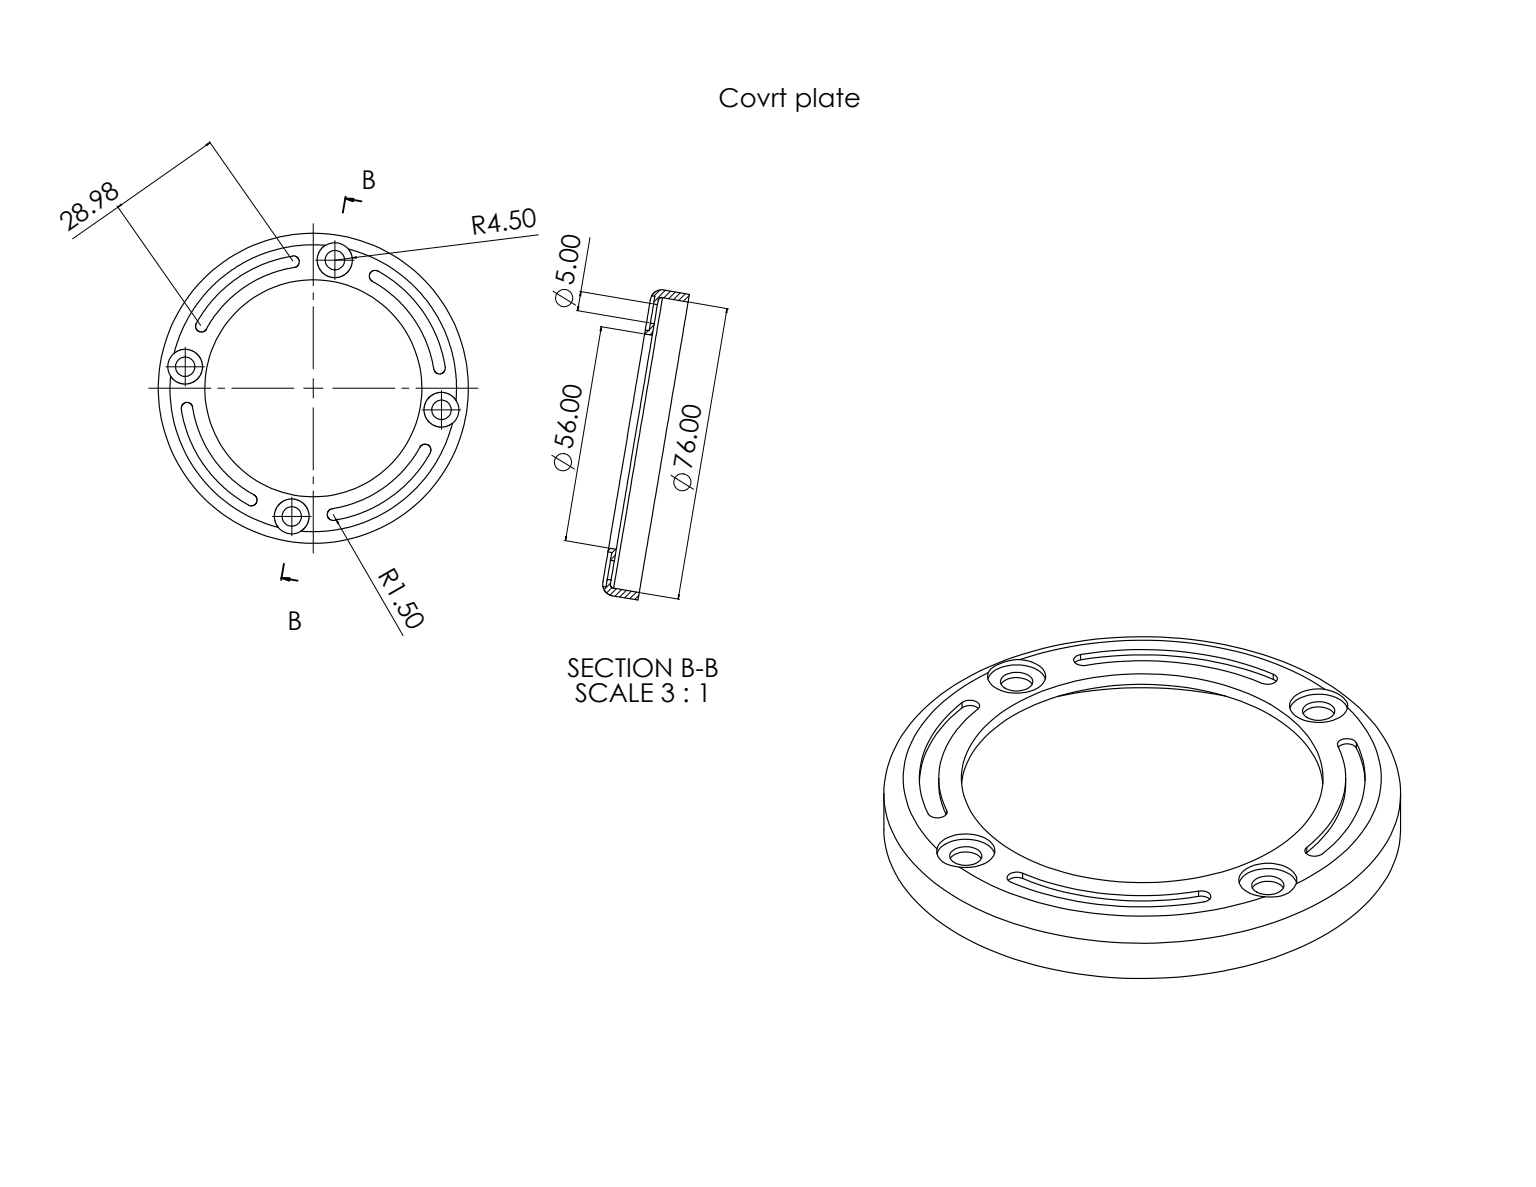
ISO-10303-21;
HEADER;
FILE_DESCRIPTION (('STEP AP214'),
    '1' );
FILE_NAME ('Covrt plate.step',
    '2026-10-19T14:05:14',
    ( '' ),
    ( '' ),
    'SwSTEP 2.0',
    'SolidWorks 2025',
    '' );
FILE_SCHEMA (( 'AUTOMOTIVE_DESIGN' ));
ENDSEC;

DATA;
#7=DIRECTION ( 'NONE',  ( 0.000000000000000000, 0.000000000000000000, 1.000000000000000000 ) ) ;
#9=ORIENTED_EDGE ( 'NONE', *, *, #8476, .T. ) ;
#15=ORIENTED_EDGE ( 'NONE', *, *, #6125, .T. ) ;
#19=DIRECTION ( 'NONE',  ( 0.000000000000000000, 0.000000000000000000, 1.000000000000000000 ) ) ;
#32=ORIENTED_EDGE ( 'NONE', *, *, #3378, .T. ) ;
#35=EDGE_CURVE ( 'NONE', #8414, #7328, #2773, .T. ) ;
#36=ORIENTED_EDGE ( 'NONE', *, *, #1808, .T. ) ;
#37=CARTESIAN_POINT ( 'NONE',  ( -7.819489076939736272, 61.89591950820473443, 36.97167050927867393 ) ) ;
#41=EDGE_CURVE ( 'NONE', #3849, #2645, #7411, .T. ) ;
#45=ORIENTED_EDGE ( 'NONE', *, *, #2688, .T. ) ;
#51=EDGE_CURVE ( 'NONE', #326, #7682, #6952, .T. ) ;
#56=CIRCLE ( 'NONE', #3832, 38.00000000000000711 ) ;
#57=EDGE_LOOP ( 'NONE', ( #2932, #7865, #7571, #5966, #8095 ) ) ;
#58=DIRECTION ( 'NONE',  ( 0.000000000000000000, 1.000000000000000000, 0.000000000000000000 ) ) ;
#64=VERTEX_POINT ( 'NONE', #213 ) ;
#66=LINE ( 'NONE', #799, #8451 ) ;
#76=AXIS2_PLACEMENT_3D ( 'NONE', #8734, #591, #7241 ) ;
#80=ORIENTED_EDGE ( 'NONE', *, *, #3650, .T. ) ;
#85=AXIS2_PLACEMENT_3D ( 'NONE', #944, #4059, #1772 ) ;
#88=ORIENTED_EDGE ( 'NONE', *, *, #8502, .F. ) ;
#89=CARTESIAN_POINT ( 'NONE',  ( 5.562309845534588959, 60.99999999999999289, -30.56426808735054479 ) ) ;
#98=CARTESIAN_POINT ( 'NONE',  ( -34.07933880998930221, 60.99999999999999289, 5.371095444502539173 ) ) ;
#116=DIRECTION ( 'NONE',  ( -0.000000000000000000, -1.000000000000000000, -0.000000000000000000 ) ) ;
#124=DIRECTION ( 'NONE',  ( 0.000000000000000000, 0.000000000000000000, 1.000000000000000000 ) ) ;
#126=CARTESIAN_POINT ( 'NONE',  ( -28.87459861216645862, 60.99999999999999289, -14.47678174684361352 ) ) ;
#129=LINE ( 'NONE', #4464, #7033 ) ;
#133=CARTESIAN_POINT ( 'NONE',  ( -5.562309845534701758, 60.99999999999999289, 33.06426808735052703 ) ) ;
#144=FACE_OUTER_BOUND ( 'NONE', #5084, .T. ) ;
#153=ORIENTED_EDGE ( 'NONE', *, *, #7147, .T. ) ;
#155=CARTESIAN_POINT ( 'NONE',  ( 37.34143203299149860, 61.94837758590841759, 4.137096292553819055 ) ) ;
#162=DIRECTION ( 'NONE',  ( 0.000000000000000000, 0.000000000000000000, 1.000000000000000000 ) ) ;
#168=FACE_OUTER_BOUND ( 'NONE', #440, .T. ) ;
#172=CIRCLE ( 'NONE', #6452, 38.00000000000000711 ) ;
#175=FACE_OUTER_BOUND ( 'NONE', #2105, .T. ) ;
#184=CARTESIAN_POINT ( 'NONE',  ( 31.11591804390324612, 60.99999999999999289, -4.904043666719942074 ) ) ;
#189=ORIENTED_EDGE ( 'NONE', *, *, #8556, .F. ) ;
#198=CIRCLE ( 'NONE', #6955, 4.500000000000005329 ) ;
#200=DIRECTION ( 'NONE',  ( 0.000000000000000000, 0.000000000000000000, 1.000000000000000000 ) ) ;
#203=DIRECTION ( 'NONE',  ( 0.000000000000000000, 0.000000000000000000, 1.000000000000000000 ) ) ;
#211=AXIS2_PLACEMENT_3D ( 'NONE', #6008, #116, #5285 ) ;
#213=CARTESIAN_POINT ( 'NONE',  ( 4.653657836759942730E-15, 52.29648987751954792, 38.00000000000000711 ) ) ;
#216=CARTESIAN_POINT ( 'NONE',  ( 3.429011037612588487E-15, 0.000000000000000000, 27.99999999999999289 ) ) ;
#222=CIRCLE ( 'NONE', #6654, 1.500000000000000888 ) ;
#224=EDGE_CURVE ( 'NONE', #6202, #6468, #9617, .T. ) ;
#225=CIRCLE ( 'NONE', #5729, 4.500000000000005329 ) ;
#239=DIRECTION ( 'NONE',  ( 0.000000000000000000, 1.000000000000000000, 0.000000000000000000 ) ) ;
#241=CARTESIAN_POINT ( 'NONE',  ( 0.000000000000000000, 60.99999999999999289, 0.000000000000000000 ) ) ;
#242=DIRECTION ( 'NONE',  ( 0.000000000000000000, 0.000000000000000000, -1.000000000000000000 ) ) ;
#245=AXIS2_PLACEMENT_3D ( 'NONE', #2886, #4538, #6229 ) ;
#246=CYLINDRICAL_SURFACE ( 'NONE', #7429, 1.500000000000001332 ) ;
#249=EDGE_CURVE ( 'NONE', #5097, #3498, #5520, .T. ) ;
#251=DIRECTION ( 'NONE',  ( 0.000000000000000000, 1.000000000000000000, 0.000000000000000000 ) ) ;
#256=ORIENTED_EDGE ( 'NONE', *, *, #2384, .T. ) ;
#258=CIRCLE ( 'NONE', #2286, 27.99999999999999289 ) ;
#259=CARTESIAN_POINT ( 'NONE',  ( -15.97678174684350871, 60.99999999999999289, 30.37459861216651191 ) ) ;
#263=LINE ( 'NONE', #7803, #7090 ) ;
#272=CARTESIAN_POINT ( 'NONE',  ( -28.87459861216645862, 60.99999999999999289, -15.97678174684361707 ) ) ;
#277=ORIENTED_EDGE ( 'NONE', *, *, #1811, .F. ) ;
#281=ORIENTED_EDGE ( 'NONE', *, *, #7582, .F. ) ;
#286=ORIENTED_EDGE ( 'NONE', *, *, #2067, .T. ) ;
#293=DIRECTION ( 'NONE',  ( -0.000000000000000000, -1.000000000000000000, -0.000000000000000000 ) ) ;
#296=ADVANCED_FACE ( 'NONE', ( #9221, #2433 ), #6373, .T. ) ;
#297=ORIENTED_EDGE ( 'NONE', *, *, #6768, .F. ) ;
#298=CARTESIAN_POINT ( 'NONE',  ( 5.137569555611264605, 61.99999999999999289, 32.59762842694627949 ) ) ;
#299=DIRECTION ( 'NONE',  ( -0.000000000000000000, 1.000000000000000000, -0.000000000000000000 ) ) ;
#304=DIRECTION ( 'NONE',  ( -0.000000000000000000, 1.000000000000000000, 0.000000000000000000 ) ) ;
#315=CARTESIAN_POINT ( 'NONE',  ( 33.06426808735054124, 60.99999999999999289, 5.562309845534586294 ) ) ;
#326=VERTEX_POINT ( 'NONE', #5646 ) ;
#331=CARTESIAN_POINT ( 'NONE',  ( 0.000000000000000000, 0.000000000000000000, 0.000000000000000000 ) ) ;
#335=EDGE_CURVE ( 'NONE', #2169, #1750, #9450, .T. ) ;
#340=DIRECTION ( 'NONE',  ( 0.000000000000000000, 1.000000000000000000, 0.000000000000000000 ) ) ;
#341=VERTEX_POINT ( 'NONE', #363 ) ;
#344=VERTEX_POINT ( 'NONE', #2620 ) ;
#345=DIRECTION ( 'NONE',  ( -0.000000000000000000, -1.000000000000000000, -0.000000000000000000 ) ) ;
#348=DIRECTION ( 'NONE',  ( 0.000000000000000000, 0.000000000000000000, 1.000000000000000000 ) ) ;
#349=CARTESIAN_POINT ( 'NONE',  ( -37.45692540970868833, 61.81802411364413530, -6.576816292457711377 ) ) ;
#350=EDGE_CURVE ( 'NONE', #3498, #6767, #2032, .T. ) ;
#353=CARTESIAN_POINT ( 'NONE',  ( 32.59762842694625817, 60.99999999999999289, -5.137569555611371186 ) ) ;
#356=ORIENTED_EDGE ( 'NONE', *, *, #480, .F. ) ;
#359=EDGE_LOOP ( 'NONE', ( #7695, #5328, #4724, #356, #5569, #5542, #45, #4880, #4061 ) ) ;
#362=CIRCLE ( 'NONE', #5560, 1.500000000000003109 ) ;
#363=CARTESIAN_POINT ( 'NONE',  ( 5.562309845534588959, 60.99999999999999289, -35.56426808735054834 ) ) ;
#366=ORIENTED_EDGE ( 'NONE', *, *, #6545, .T. ) ;
#368=DIRECTION ( 'NONE',  ( 0.000000000000000000, 0.000000000000000000, -1.000000000000000000 ) ) ;
#372=CIRCLE ( 'NONE', #1158, 34.49999999999998579 ) ;
#373=ADVANCED_FACE ( 'NONE', ( #4991, #2055, #5082, #4350, #4442, #6692 ), #1522, .T. ) ;
#376=CARTESIAN_POINT ( 'NONE',  ( -33.06426808735054124, 60.99999999999999289, -8.062309845534585406 ) ) ;
#377=ORIENTED_EDGE ( 'NONE', *, *, #4261, .T. ) ;
#383=FACE_OUTER_BOUND ( 'NONE', #9081, .T. ) ;
#385=DIRECTION ( 'NONE',  ( 0.000000000000000000, -1.000000000000000000, 0.000000000000000000 ) ) ;
#387=ORIENTED_EDGE ( 'NONE', *, *, #7583, .F. ) ;
#388=VECTOR ( 'NONE', #3945, 1000.000000000000000 ) ;
#390=DIRECTION ( 'NONE',  ( -0.000000000000000000, 1.000000000000000000, 0.000000000000000000 ) ) ;
#392=CARTESIAN_POINT ( 'NONE',  ( 5.562309845534932684, 61.83753588906734677, -37.56426808735049150 ) ) ;
#400=CARTESIAN_POINT ( 'NONE',  ( -37.52916669695763119, 61.87792984901915361, -4.938418073206593206 ) ) ;
#402=ORIENTED_EDGE ( 'NONE', *, *, #8610, .F. ) ;
#411=EDGE_CURVE ( 'NONE', #4511, #7590, #7183, .T. ) ;
#424=ORIENTED_EDGE ( 'NONE', *, *, #837, .F. ) ;
#426=AXIS2_PLACEMENT_3D ( 'NONE', #882, #3183, #242 ) ;
#429=CIRCLE ( 'NONE', #5919, 34.49999999999998579 ) ;
#431=ADVANCED_FACE ( 'NONE', ( #676 ), #2230, .F. ) ;
#433=CYLINDRICAL_SURFACE ( 'NONE', #5292, 4.500000000000003553 ) ;
#435=CIRCLE ( 'NONE', #6247, 1.500000000000003109 ) ;
#440=EDGE_LOOP ( 'NONE', ( #9334, #387, #3842, #4081 ) ) ;
#444=CARTESIAN_POINT ( 'NONE',  ( 0.000000000000000000, 61.99999999999999289, 0.000000000000000000 ) ) ;
#447=DIRECTION ( 'NONE',  ( -0.000000000000000000, 1.000000000000000000, -0.000000000000000000 ) ) ;
#449=EDGE_LOOP ( 'NONE', ( #4120, #8855, #5186, #6580 ) ) ;
#453=DIRECTION ( 'NONE',  ( 0.000000000000000000, 0.000000000000000000, -1.000000000000000000 ) ) ;
#455=DIRECTION ( 'NONE',  ( 0.000000000000000000, 1.000000000000000000, 0.000000000000000000 ) ) ;
#457=DIRECTION ( 'NONE',  ( 0.000000000000000000, 0.000000000000000000, -1.000000000000000000 ) ) ;
#459=ORIENTED_EDGE ( 'NONE', *, *, #1954, .T. ) ;
#465=( NAMED_UNIT ( * ) PLANE_ANGLE_UNIT ( ) SI_UNIT ( $, .RADIAN. ) );
#476=DIRECTION ( 'NONE',  ( -1.224646799147354440E-16, 0.000000000000000000, -1.000000000000000000 ) ) ;
#477=AXIS2_PLACEMENT_3D ( 'NONE', #8724, #3437, #4921 ) ;
#480=EDGE_CURVE ( 'NONE', #2405, #7052, #1136, .T. ) ;
#491=DIRECTION ( 'NONE',  ( 0.000000000000000000, 0.000000000000000000, 1.000000000000000000 ) ) ;
#499=DIRECTION ( 'NONE',  ( 0.000000000000000000, 0.000000000000000000, 1.000000000000000000 ) ) ;
#502=FACE_BOUND ( 'NONE', #5683, .T. ) ;
#506=CARTESIAN_POINT ( 'NONE',  ( 30.18708036726505028, 60.99999999999999289, 16.70299909897265778 ) ) ;
#510=ADVANCED_FACE ( 'NONE', ( #144 ), #7240, .F. ) ;
#512=VECTOR ( 'NONE', #9362, 1000.000000000000000 ) ;
#523=AXIS2_PLACEMENT_3D ( 'NONE', #9479, #3779, #453 ) ;
#525=DIRECTION ( 'NONE',  ( 0.000000000000000000, 1.000000000000000000, 0.000000000000000000 ) ) ;
#526=EDGE_CURVE ( 'NONE', #1263, #8611, #8767, .T. ) ;
#537=CARTESIAN_POINT ( 'NONE',  ( 33.06426808735054124, 60.99999999999999289, 10.06230984553459251 ) ) ;
#543=EDGE_LOOP ( 'NONE', ( #1051, #1882 ) ) ;
#552=CARTESIAN_POINT ( 'NONE',  ( 0.000000000000000000, 60.99999999999999289, 0.000000000000000000 ) ) ;
#567=CARTESIAN_POINT ( 'NONE',  ( 0.000000000000000000, 52.29648987751954792, -38.00000000000000711 ) ) ;
#582=CARTESIAN_POINT ( 'NONE',  ( 0.000000000000000000, 60.99999999999999289, 0.000000000000000000 ) ) ;
#583=DIRECTION ( 'NONE',  ( 0.000000000000000000, 0.000000000000000000, -1.000000000000000000 ) ) ;
#584=CIRCLE ( 'NONE', #9564, 2.500000000000002220 ) ;
#591=DIRECTION ( 'NONE',  ( 0.000000000000000000, 1.000000000000000000, 0.000000000000000000 ) ) ;
#594=CARTESIAN_POINT ( 'NONE',  ( -4.904043666719616112, 61.99999999999999289, -31.11591804390330651 ) ) ;
#612=PLANE ( 'NONE',  #732 ) ;
#613=ORIENTED_EDGE ( 'NONE', *, *, #7697, .F. ) ;
#617=EDGE_LOOP ( 'NONE', ( #366, #613, #1994, #8826 ) ) ;
#618=CARTESIAN_POINT ( 'NONE',  ( -16.70299909897276081, 61.99999999999999289, 30.18708036726496857 ) ) ;
#630=DIRECTION ( 'NONE',  ( 0.000000000000000000, 1.000000000000000000, 0.000000000000000000 ) ) ;
#632=AXIS2_PLACEMENT_3D ( 'NONE', #9012, #5209, #2137 ) ;
#637=AXIS2_PLACEMENT_3D ( 'NONE', #6190, #2432, #823 ) ;
#639=CARTESIAN_POINT ( 'NONE',  ( 0.000000000000000000, 52.29648987751954792, -40.00000000000000711 ) ) ;
#670=DIRECTION ( 'NONE',  ( 0.000000000000000000, 0.000000000000000000, 1.000000000000000000 ) ) ;
#671=AXIS2_PLACEMENT_3D ( 'NONE', #7509, #58, #2953 ) ;
#673=AXIS2_PLACEMENT_3D ( 'NONE', #8739, #2698, #4205 ) ;
#675=ORIENTED_EDGE ( 'NONE', *, *, #3911, .F. ) ;
#676=FACE_OUTER_BOUND ( 'NONE', #8642, .T. ) ;
#678=DIRECTION ( 'NONE',  ( -0.000000000000000000, 1.000000000000000000, -0.000000000000000000 ) ) ;
#679=CARTESIAN_POINT ( 'NONE',  ( -32.59762842694629370, 61.99999999999999289, 5.137569555611143812 ) ) ;
#692=DIRECTION ( 'NONE',  ( 0.000000000000000000, 1.000000000000000000, 0.000000000000000000 ) ) ;
#695=ORIENTED_EDGE ( 'NONE', *, *, #6119, .T. ) ;
#699=CIRCLE ( 'NONE', #1016, 4.500000000000005329 ) ;
#703=ORIENTED_EDGE ( 'NONE', *, *, #1808, .F. ) ;
#707=DIRECTION ( 'NONE',  ( 0.000000000000000000, 0.000000000000000000, -1.000000000000000000 ) ) ;
#727=AXIS2_PLACEMENT_3D ( 'NONE', #6622, #9643, #2128 ) ;
#731=DIRECTION ( 'NONE',  ( 0.000000000000000000, 0.000000000000000000, 1.000000000000000000 ) ) ;
#732=AXIS2_PLACEMENT_3D ( 'NONE', #5881, #2122, #3614 ) ;
#740=DIRECTION ( 'NONE',  ( -0.000000000000000000, 1.000000000000000000, -0.000000000000000000 ) ) ;
#747=ORIENTED_EDGE ( 'NONE', *, *, #8375, .F. ) ;
#749=EDGE_CURVE ( 'NONE', #4632, #7580, #3329, .T. ) ;
#752=DIRECTION ( 'NONE',  ( 0.000000000000000000, 1.000000000000000000, 0.000000000000000000 ) ) ;
#753=DIRECTION ( 'NONE',  ( -0.000000000000000000, 1.000000000000000000, -0.000000000000000000 ) ) ;
#763=ORIENTED_EDGE ( 'NONE', *, *, #7205, .T. ) ;
#765=ORIENTED_EDGE ( 'NONE', *, *, #4331, .T. ) ;
#766=ORIENTED_EDGE ( 'NONE', *, *, #2477, .T. ) ;
#769=FACE_OUTER_BOUND ( 'NONE', #3306, .T. ) ;
#772=ORIENTED_EDGE ( 'NONE', *, *, #7387, .T. ) ;
#775=CARTESIAN_POINT ( 'NONE',  ( -7.214865095667844841, 61.84561525624321376, 37.26328141369679514 ) ) ;
#786=PRODUCT ( 'Covrt plate', 'Covrt plate', '', ( #2257 ) ) ;
#792=CARTESIAN_POINT ( 'NONE',  ( 5.137569555611264605, 60.99999999999999289, 32.59762842694627949 ) ) ;
#795=CARTESIAN_POINT ( 'NONE',  ( 0.000000000000000000, 61.99999999999999289, 0.000000000000000000 ) ) ;
#796=ORIENTED_EDGE ( 'NONE', *, *, #224, .F. ) ;
#799=CARTESIAN_POINT ( 'NONE',  ( 5.371095444502685723, 60.99999999999999289, 34.07933880998929510 ) ) ;
#802=DIRECTION ( 'NONE',  ( -0.000000000000000000, 1.000000000000000000, -0.000000000000000000 ) ) ;
#804=ORIENTED_EDGE ( 'NONE', *, *, #7649, .F. ) ;
#807=CARTESIAN_POINT ( 'NONE',  ( 32.59762842694625817, 61.99999999999999289, -3.637569555611369854 ) ) ;
#823=DIRECTION ( 'NONE',  ( 0.000000000000000000, 0.000000000000000000, 1.000000000000000000 ) ) ;
#830=FACE_OUTER_BOUND ( 'NONE', #8162, .T. ) ;
#837=EDGE_CURVE ( 'NONE', #7858, #6645, #2417, .T. ) ;
#838=DIRECTION ( 'NONE',  ( 0.000000000000000000, 0.000000000000000000, 1.000000000000000000 ) ) ;
#845=CIRCLE ( 'NONE', #8729, 40.00000000000000711 ) ;
#846=ORIENTED_EDGE ( 'NONE', *, *, #9159, .F. ) ;
#849=VERTEX_POINT ( 'NONE', #6339 ) ;
#850=PRODUCT_DEFINITION ( 'UNKNOWN', '', #5853, #3314 ) ;
#853=ORIENTED_EDGE ( 'NONE', *, *, #1832, .F. ) ;
#856=ORIENTED_EDGE ( 'NONE', *, *, #5980, .T. ) ;
#857=CARTESIAN_POINT ( 'NONE',  ( 0.000000000000000000, 60.99999999999999289, 0.000000000000000000 ) ) ;
#860=PLANE ( 'NONE',  #9656 ) ;
#861=DIRECTION ( 'NONE',  ( 0.000000000000000000, 0.000000000000000000, 1.000000000000000000 ) ) ;
#882=CARTESIAN_POINT ( 'NONE',  ( 5.562309845534588959, 69.99999999999998579, -33.06426808735054124 ) ) ;
#884=DIRECTION ( 'NONE',  ( 0.000000000000000000, -0.000000000000000000, 1.000000000000000000 ) ) ;
#886=DIRECTION ( 'NONE',  ( -0.000000000000000000, 1.000000000000000000, -0.000000000000000000 ) ) ;
#889=EDGE_CURVE ( 'NONE', #7059, #4514, #9064, .T. ) ;
#896=DIRECTION ( 'NONE',  ( 0.000000000000000000, 0.000000000000000000, 1.000000000000000000 ) ) ;
#901=CARTESIAN_POINT ( 'NONE',  ( 33.06426808735054124, 69.99999999999998579, 8.062309845534588959 ) ) ;
#903=VERTEX_POINT ( 'NONE', #9505 ) ;
#904=DIRECTION ( 'NONE',  ( -0.000000000000000000, 1.000000000000000000, -0.000000000000000000 ) ) ;
#914=ORIENTED_EDGE ( 'NONE', *, *, #2519, .F. ) ;
#922=EDGE_LOOP ( 'NONE', ( #3656, #1162 ) ) ;
#934=CARTESIAN_POINT ( 'NONE',  ( 37.38678512219217254, 61.82631808411006347, 6.843790051325325585 ) ) ;
#935=ORIENTED_EDGE ( 'NONE', *, *, #2688, .F. ) ;
#938=DIRECTION ( 'NONE',  ( 0.000000000000000000, 0.000000000000000000, 1.000000000000000000 ) ) ;
#944=CARTESIAN_POINT ( 'NONE',  ( 0.000000000000000000, 60.99999999999999289, 0.000000000000000000 ) ) ;
#946=DIRECTION ( 'NONE',  ( -0.000000000000000000, 1.000000000000000000, -0.000000000000000000 ) ) ;
#949=ORIENTED_EDGE ( 'NONE', *, *, #7446, .F. ) ;
#957=DIRECTION ( 'NONE',  ( 0.000000000000000000, 0.000000000000000000, -1.000000000000000000 ) ) ;
#974=CARTESIAN_POINT ( 'NONE',  ( -27.56211685706797709, 60.99999999999999289, -15.25056439471436676 ) ) ;
#976=AXIS2_PLACEMENT_3D ( 'NONE', #7526, #1546, #19 ) ;
#980=CARTESIAN_POINT ( 'NONE',  ( -5.562309845534701758, 60.99999999999999289, 33.06426808735052703 ) ) ;
#981=CARTESIAN_POINT ( 'NONE',  ( 37.56827137616963341, 61.82639507982414528, 5.763559184779289524 ) ) ;
#991=EDGE_CURVE ( 'NONE', #6002, #8252, #1567, .T. ) ;
#1002=EDGE_LOOP ( 'NONE', ( #5300, #5992, #7430, #4313 ) ) ;
#1016=AXIS2_PLACEMENT_3D ( 'NONE', #5940, #6582, #8962 ) ;
#1019=FACE_OUTER_BOUND ( 'NONE', #9246, .T. ) ;
#1028=ORIENTED_EDGE ( 'NONE', *, *, #41, .F. ) ;
#1035=DIRECTION ( 'NONE',  ( -0.000000000000000000, -1.000000000000000000, -0.000000000000000000 ) ) ;
#1050=VECTOR ( 'NONE', #7003, 1000.000000000000000 ) ;
#1051=ORIENTED_EDGE ( 'NONE', *, *, #2670, .F. ) ;
#1052=CARTESIAN_POINT ( 'NONE',  ( -33.06426808735054124, 59.99999999999999289, -8.062309845534585406 ) ) ;
#1053=ORIENTED_EDGE ( 'NONE', *, *, #1905, .F. ) ;
#1060=CARTESIAN_POINT ( 'NONE',  ( 5.562309845534932684, 61.99999999999999289, -33.06426808735049150 ) ) ;
#1061=EDGE_CURVE ( 'NONE', #5641, #1736, #225, .T. ) ;
#1062=CARTESIAN_POINT ( 'NONE',  ( -30.18708036726492594, 61.99999999999999289, -16.70299909897287094 ) ) ;
#1063=EDGE_LOOP ( 'NONE', ( #4155, #7732, #4121, #7579 ) ) ;
#1067=CARTESIAN_POINT ( 'NONE',  ( -34.07933880998930221, 60.99999999999999289, 5.371095444502539173 ) ) ;
#1072=DIRECTION ( 'NONE',  ( -0.000000000000000000, 1.000000000000000000, -0.000000000000000000 ) ) ;
#1087=CARTESIAN_POINT ( 'NONE',  ( 0.000000000000000000, 0.000000000000000000, -40.00000000000000711 ) ) ;
#1090=CARTESIAN_POINT ( 'NONE',  ( 0.000000000000000000, 60.99999999999999289, 0.000000000000000000 ) ) ;
#1101=VERTEX_POINT ( 'NONE', #3341 ) ;
#1122=AXIS2_PLACEMENT_3D ( 'NONE', #6934, #3989, #884 ) ;
#1123=CARTESIAN_POINT ( 'NONE',  ( 3.429011037612588487E-15, 61.99999999999999289, 27.99999999999999289 ) ) ;
#1126=EDGE_CURVE ( 'NONE', #5694, #5111, #7904, .T. ) ;
#1129=LINE ( 'NONE', #4932, #3212 ) ;
#1130=ORIENTED_EDGE ( 'NONE', *, *, #2017, .F. ) ;
#1131=DIRECTION ( 'NONE',  ( -1.000000000000000000, 0.000000000000000000, -3.491481338843133355E-15 ) ) ;
#1134=LINE ( 'NONE', #4292, #1183 ) ;
#1136=B_SPLINE_CURVE_WITH_KNOTS ( 'NONE', 3,
 ( #7546, #5900, #4584, #8927, #37, #775, #3785, #7393, #7591, #2145 ),
 .UNSPECIFIED., .F., .F.,
 ( 4, 2, 2, 2, 4 ),
 ( 0.003057178249550608282, 0.004067793317122878408, 0.005078408384695147666, 0.006089023452267415190, 0.007099638519839682714 ),
 .UNSPECIFIED. ) ;
#1137=CARTESIAN_POINT ( 'NONE',  ( -37.56827137616963341, 61.82639507982414528, -5.763559184779289524 ) ) ;
#1138=CARTESIAN_POINT ( 'NONE',  ( 0.000000000000000000, 59.99999999999999289, -37.00000000000000711 ) ) ;
#1139=VERTEX_POINT ( 'NONE', #2110 ) ;
#1140=CARTESIAN_POINT ( 'NONE',  ( 0.000000000000000000, 60.99999999999999289, 0.000000000000000000 ) ) ;
#1158=AXIS2_PLACEMENT_3D ( 'NONE', #6526, #525, #3520 ) ;
#1159=AXIS2_PLACEMENT_3D ( 'NONE', #2694, #1911, #3593 ) ;
#1162=ORIENTED_EDGE ( 'NONE', *, *, #7492, .F. ) ;
#1163=CARTESIAN_POINT ( 'NONE',  ( 15.97678174684330799, 61.99999999999999289, -28.87459861216662205 ) ) ;
#1169=DIRECTION ( 'NONE',  ( -0.000000000000000000, 1.000000000000000000, -0.000000000000000000 ) ) ;
#1170=CARTESIAN_POINT ( 'NONE',  ( -16.70299909897276081, 60.99999999999999289, 30.18708036726496857 ) ) ;
#1183=VECTOR ( 'NONE', #345, 1000.000000000000000 ) ;
#1191=FACE_OUTER_BOUND ( 'NONE', #5726, .T. ) ;
#1198=TOROIDAL_SURFACE ( 'NONE', #1669, 37.00000000000000711, 3.000000000000002665 ) ;
#1200=CIRCLE ( 'NONE', #4675, 1.500000000000000888 ) ;
#1206=ORIENTED_EDGE ( 'NONE', *, *, #5319, .F. ) ;
#1216=DIRECTION ( 'NONE',  ( 0.000000000000000000, 0.000000000000000000, 1.000000000000000000 ) ) ;
#1218=ORIENTED_EDGE ( 'NONE', *, *, #2424, .T. ) ;
#1236=CARTESIAN_POINT ( 'NONE',  ( -33.06426808735054124, 60.99999999999999289, -10.06230984553459251 ) ) ;
#1239=LINE ( 'NONE', #9623, #9208 ) ;
#1241=EDGE_CURVE ( 'NONE', #7328, #5641, #699, .T. ) ;
#1244=DIRECTION ( 'NONE',  ( -0.000000000000000000, 1.000000000000000000, -0.000000000000000000 ) ) ;
#1247=ORIENTED_EDGE ( 'NONE', *, *, #6944, .T. ) ;
#1248=DIRECTION ( 'NONE',  ( 0.000000000000000000, 0.000000000000000000, 1.000000000000000000 ) ) ;
#1252=VERTEX_POINT ( 'NONE', #618 ) ;
#1254=ADVANCED_FACE ( 'NONE', ( #7431 ), #5844, .F. ) ;
#1259=VECTOR ( 'NONE', #7731, 1000.000000000000000 ) ;
#1263=VERTEX_POINT ( 'NONE', #5939 ) ;
#1267=DIRECTION ( 'NONE',  ( 0.000000000000000000, 0.000000000000000000, -1.000000000000000000 ) ) ;
#1269=AXIS2_PLACEMENT_3D ( 'NONE', #7980, #1851, #9267 ) ;
#1274=VECTOR ( 'NONE', #1169, 1000.000000000000000 ) ;
#1295=CARTESIAN_POINT ( 'NONE',  ( 0.000000000000000000, 61.99999999999999289, -27.99999999999999289 ) ) ;
#1299=PLANE ( 'NONE',  #6702 ) ;
#1305=EDGE_CURVE ( 'NONE', #7141, #1519, #8622, .T. ) ;
#1306=ADVANCED_FACE ( 'NONE', ( #1357 ), #7276, .F. ) ;
#1311=ORIENTED_EDGE ( 'NONE', *, *, #3040, .T. ) ;
#1318=AXIS2_PLACEMENT_3D ( 'NONE', #3163, #4618, #861 ) ;
#1327=VECTOR ( 'NONE', #3797, 1000.000000000000000 ) ;
#1339=AXIS2_PLACEMENT_3D ( 'NONE', #1090, #6316, #9337 ) ;
#1341=ORIENTED_EDGE ( 'NONE', *, *, #9122, .T. ) ;
#1343=ORIENTED_EDGE ( 'NONE', *, *, #8556, .T. ) ;
#1348=VECTOR ( 'NONE', #2407, 1000.000000000000000 ) ;
#1350=AXIS2_PLACEMENT_3D ( 'NONE', #2273, #5311, #1644 ) ;
#1351=VECTOR ( 'NONE', #678, 1000.000000000000000 ) ;
#1353=AXIS2_PLACEMENT_3D ( 'NONE', #3373, #4912, #4229 ) ;
#1356=VERTEX_POINT ( 'NONE', #8072 ) ;
#1357=FACE_OUTER_BOUND ( 'NONE', #4149, .T. ) ;
#1366=CARTESIAN_POINT ( 'NONE',  ( 5.562309845534588959, 69.99999999999998579, -35.56426808735054834 ) ) ;
#1368=ORIENTED_EDGE ( 'NONE', *, *, #7402, .F. ) ;
#1369=DIRECTION ( 'NONE',  ( 0.000000000000000000, 1.000000000000000000, 0.000000000000000000 ) ) ;
#1371=DIRECTION ( 'NONE',  ( 0.000000000000000000, 1.000000000000000000, 0.000000000000000000 ) ) ;
#1386=EDGE_CURVE ( 'NONE', #3246, #2405, #6540, .T. ) ;
#1388=ORIENTED_EDGE ( 'NONE', *, *, #9343, .F. ) ;
#1392=EDGE_LOOP ( 'NONE', ( #772, #8170, #5356, #7756, #5921 ) ) ;
#1399=ORIENTED_EDGE ( 'NONE', *, *, #1725, .T. ) ;
#1401=ORIENTED_EDGE ( 'NONE', *, *, #6490, .F. ) ;
#1403=FACE_OUTER_BOUND ( 'NONE', #5650, .T. ) ;
#1405=DIRECTION ( 'NONE',  ( -0.000000000000000000, 1.000000000000000000, -0.000000000000000000 ) ) ;
#1412=CARTESIAN_POINT ( 'NONE',  ( -34.07933880998930221, 61.99999999999999289, 5.371095444502539173 ) ) ;
#1432=VERTEX_POINT ( 'NONE', #3874 ) ;
#1435=EDGE_LOOP ( 'NONE', ( #8983, #8517, #7630, #6035 ) ) ;
#1436=DIRECTION ( 'NONE',  ( 0.000000000000000000, -1.000000000000000000, 0.000000000000000000 ) ) ;
#1444=CARTESIAN_POINT ( 'NONE',  ( -33.06426808735054124, 60.99999999999999289, -3.062309845534580077 ) ) ;
#1450=DIRECTION ( 'NONE',  ( 0.000000000000000000, 0.000000000000000000, -1.000000000000000000 ) ) ;
#1458=DIRECTION ( 'NONE',  ( 0.000000000000000000, 1.000000000000000000, 0.000000000000000000 ) ) ;
#1466=CARTESIAN_POINT ( 'NONE',  ( 0.000000000000000000, 61.99999999999999289, 0.000000000000000000 ) ) ;
#1469=CARTESIAN_POINT ( 'NONE',  ( -28.87459861216645862, 60.99999999999999289, -15.97678174684361707 ) ) ;
#1472=ADVANCED_FACE ( 'NONE', ( #4524 ), #7680, .F. ) ;
#1474=DIRECTION ( 'NONE',  ( 0.000000000000000000, 1.000000000000000000, 0.000000000000000000 ) ) ;
#1475=CYLINDRICAL_SURFACE ( 'NONE', #8450, 1.500000000000000888 ) ;
#1476=ORIENTED_EDGE ( 'NONE', *, *, #6421, .T. ) ;
#1479=CARTESIAN_POINT ( 'NONE',  ( -33.06426808735054124, 61.99999999999999289, -5.562309845534586294 ) ) ;
#1498=VERTEX_POINT ( 'NONE', #1052 ) ;
#1499=CARTESIAN_POINT ( 'NONE',  ( -33.06426808735054124, 61.99999999999999289, -5.562309845534586294 ) ) ;
#1500=AXIS2_PLACEMENT_3D ( 'NONE', #2870, #8858, #6668 ) ;
#1506=VECTOR ( 'NONE', #1244, 1000.000000000000000 ) ;
#1507=AXIS2_PLACEMENT_3D ( 'NONE', #6375, #4856, #7920 ) ;
#1509=ADVANCED_FACE ( 'NONE', ( #1840 ), #5771, .T. ) ;
#1515=EDGE_CURVE ( 'NONE', #4632, #1356, #2598, .T. ) ;
#1519=VERTEX_POINT ( 'NONE', #8613 ) ;
#1522=PLANE ( 'NONE',  #3401 ) ;
#1528=ADVANCED_FACE ( 'NONE', ( #3970 ), #3263, .F. ) ;
#1529=FACE_OUTER_BOUND ( 'NONE', #5875, .T. ) ;
#1531=ORIENTED_EDGE ( 'NONE', *, *, #5980, .F. ) ;
#1536=VERTEX_POINT ( 'NONE', #7167 ) ;
#1546=DIRECTION ( 'NONE',  ( 0.000000000000000000, 1.000000000000000000, 0.000000000000000000 ) ) ;
#1555=ORIENTED_EDGE ( 'NONE', *, *, #5644, .T. ) ;
#1559=ORIENTED_EDGE ( 'NONE', *, *, #2067, .F. ) ;
#1567=CIRCLE ( 'NONE', #2813, 1.500000000000001332 ) ;
#1568=DIRECTION ( 'NONE',  ( 0.000000000000000000, 0.000000000000000000, 1.000000000000000000 ) ) ;
#1590=FACE_OUTER_BOUND ( 'NONE', #4470, .T. ) ;
#1598=CARTESIAN_POINT ( 'NONE',  ( 4.904043666719842598, 61.99999999999999289, 31.11591804390326743 ) ) ;
#1608=ADVANCED_FACE ( 'NONE', ( #2770 ), #8802, .F. ) ;
#1609=EDGE_CURVE ( 'NONE', #5153, #1498, #3549, .T. ) ;
#1610=LINE ( 'NONE', #184, #5250 ) ;
#1613=EDGE_LOOP ( 'NONE', ( #3161, #8396 ) ) ;
#1615=CIRCLE ( 'NONE', #8233, 40.00000000000000711 ) ;
#1623=DIRECTION ( 'NONE',  ( 0.000000000000000000, 0.000000000000000000, 1.000000000000000000 ) ) ;
#1628=CIRCLE ( 'NONE', #7297, 1.500000000000001332 ) ;
#1629=ORIENTED_EDGE ( 'NONE', *, *, #5644, .F. ) ;
#1630=CARTESIAN_POINT ( 'NONE',  ( -15.97678174684350871, 61.99999999999999289, 28.87459861216650836 ) ) ;
#1638=DIRECTION ( 'NONE',  ( 0.000000000000000000, -1.000000000000000000, 0.000000000000000000 ) ) ;
#1639=VERTEX_POINT ( 'NONE', #7966 ) ;
#1640=DIRECTION ( 'NONE',  ( -0.000000000000000000, -1.000000000000000000, -0.000000000000000000 ) ) ;
#1641=CYLINDRICAL_SURFACE ( 'NONE', #1783, 4.500000000000003553 ) ;
#1643=ORIENTED_EDGE ( 'NONE', *, *, #1775, .T. ) ;
#1644=DIRECTION ( 'NONE',  ( 0.000000000000000000, 0.000000000000000000, 1.000000000000000000 ) ) ;
#1646=ORIENTED_EDGE ( 'NONE', *, *, #6791, .F. ) ;
#1650=CARTESIAN_POINT ( 'NONE',  ( 33.06426808735054124, 60.99999999999999289, 8.062309845534588959 ) ) ;
#1665=VERTEX_POINT ( 'NONE', #1295 ) ;
#1669=AXIS2_PLACEMENT_3D ( 'NONE', #7593, #4434, #3685 ) ;
#1678=DIRECTION ( 'NONE',  ( 0.000000000000000000, 0.000000000000000000, -1.000000000000000000 ) ) ;
#1684=ORIENTED_EDGE ( 'NONE', *, *, #4456, .F. ) ;
#1691=DIRECTION ( 'NONE',  ( 0.000000000000000000, 0.000000000000000000, 1.000000000000000000 ) ) ;
#1695=CARTESIAN_POINT ( 'NONE',  ( -5.134502662544168317, 61.85904243767789978, 37.56426808735054124 ) ) ;
#1699=ORIENTED_EDGE ( 'NONE', *, *, #7492, .T. ) ;
#1703=ORIENTED_EDGE ( 'NONE', *, *, #335, .T. ) ;
#1705=CARTESIAN_POINT ( 'NONE',  ( 5.562309845534932684, 60.99999999999999289, -33.06426808735049150 ) ) ;
#1710=CARTESIAN_POINT ( 'NONE',  ( 28.87459861216657231, 60.99999999999999289, 15.97678174684340924 ) ) ;
#1711=CARTESIAN_POINT ( 'NONE',  ( 28.87459861216657231, 60.99999999999999289, 15.97678174684340924 ) ) ;
#1713=CYLINDRICAL_SURFACE ( 'NONE', #9378, 4.500000000000004441 ) ;
#1720=CARTESIAN_POINT ( 'NONE',  ( 36.80315167070719440, 61.92350945662830952, 8.081333402833552171 ) ) ;
#1725=EDGE_CURVE ( 'NONE', #9714, #1263, #66, .T. ) ;
#1726=CARTESIAN_POINT ( 'NONE',  ( 5.562309845534933572, 60.99999999999999289, -37.56426808735049150 ) ) ;
#1727=ORIENTED_EDGE ( 'NONE', *, *, #8490, .T. ) ;
#1734=DIRECTION ( 'NONE',  ( 0.000000000000000000, 1.000000000000000000, 0.000000000000000000 ) ) ;
#1736=VERTEX_POINT ( 'NONE', #7517 ) ;
#1740=CIRCLE ( 'NONE', #6774, 4.500000000000004441 ) ;
#1749=DIRECTION ( 'NONE',  ( -0.000000000000000000, -1.000000000000000000, -0.000000000000000000 ) ) ;
#1750=VERTEX_POINT ( 'NONE', #6164 ) ;
#1764=DIRECTION ( 'NONE',  ( -1.000000000000000000, 0.000000000000000000, 0.000000000000000000 ) ) ;
#1766=CIRCLE ( 'NONE', #7287, 1.500000000000001332 ) ;
#1767=CARTESIAN_POINT ( 'NONE',  ( 0.000000000000000000, 52.29648987751954792, -38.00000000000000711 ) ) ;
#1772=DIRECTION ( 'NONE',  ( 0.000000000000000000, 0.000000000000000000, 1.000000000000000000 ) ) ;
#1773=VECTOR ( 'NONE', #2596, 1000.000000000000000 ) ;
#1775=EDGE_CURVE ( 'NONE', #4511, #1139, #9103, .T. ) ;
#1778=ORIENTED_EDGE ( 'NONE', *, *, #5924, .T. ) ;
#1781=EDGE_LOOP ( 'NONE', ( #1206, #1555, #8468, #4358 ) ) ;
#1782=DIRECTION ( 'NONE',  ( 0.000000000000000000, -1.000000000000000000, 0.000000000000000000 ) ) ;
#1783=AXIS2_PLACEMENT_3D ( 'NONE', #133, #5403, #8363 ) ;
#1784=CARTESIAN_POINT ( 'NONE',  ( 5.562309845534932684, 60.99999999999999289, -33.06426808735049150 ) ) ;
#1808=EDGE_CURVE ( 'NONE', #8204, #4254, #2929, .T. ) ;
#1811=EDGE_CURVE ( 'NONE', #3433, #4254, #4460, .T. ) ;
#1815=ORIENTED_EDGE ( 'NONE', *, *, #3378, .F. ) ;
#1820=AXIS2_PLACEMENT_3D ( 'NONE', #6636, #3787, #8929 ) ;
#1825=VECTOR ( 'NONE', #4108, 1000.000000000000000 ) ;
#1832=EDGE_CURVE ( 'NONE', #1139, #1536, #8620, .T. ) ;
#1840=FACE_OUTER_BOUND ( 'NONE', #5673, .T. ) ;
#1846=CARTESIAN_POINT ( 'NONE',  ( 32.59762842694625817, 61.99999999999999289, -5.137569555611371186 ) ) ;
#1849=ADVANCED_FACE ( 'NONE', ( #1590 ), #3106, .F. ) ;
#1851=DIRECTION ( 'NONE',  ( -0.000000000000000000, -1.000000000000000000, -0.000000000000000000 ) ) ;
#1854=FACE_BOUND ( 'NONE', #8943, .T. ) ;
#1862=CARTESIAN_POINT ( 'NONE',  ( 8.634329568050956638, 61.97962948615073486, -36.36986309197408218 ) ) ;
#1866=CARTESIAN_POINT ( 'NONE',  ( 36.86535760663189620, 61.99999999999999289, 3.153634179030289530 ) ) ;
#1872=LINE ( 'NONE', #4008, #1050 ) ;
#1879=CARTESIAN_POINT ( 'NONE',  ( 32.59762842694625817, 61.99999999999999289, -5.137569555611371186 ) ) ;
#1880=ORIENTED_EDGE ( 'NONE', *, *, #9032, .T. ) ;
#1882=ORIENTED_EDGE ( 'NONE', *, *, #9537, .F. ) ;
#1889=FACE_OUTER_BOUND ( 'NONE', #2046, .T. ) ;
#1899=AXIS2_PLACEMENT_3D ( 'NONE', #2856, #3561, #2064 ) ;
#1903=DIRECTION ( 'NONE',  ( 0.000000000000000000, -1.000000000000000000, 0.000000000000000000 ) ) ;
#1905=EDGE_CURVE ( 'NONE', #9543, #6002, #429, .T. ) ;
#1911=DIRECTION ( 'NONE',  ( 0.000000000000000000, 1.000000000000000000, 0.000000000000000000 ) ) ;
#1932=DIRECTION ( 'NONE',  ( -0.000000000000000000, -1.000000000000000000, -0.000000000000000000 ) ) ;
#1934=ADVANCED_FACE ( 'NONE', ( #3408 ), #5495, .F. ) ;
#1938=CIRCLE ( 'NONE', #7623, 2.499999999999998668 ) ;
#1947=EDGE_CURVE ( 'NONE', #5164, #2072, #7908, .T. ) ;
#1949=CARTESIAN_POINT ( 'NONE',  ( 5.137569555611264605, 61.99999999999999289, 32.59762842694627949 ) ) ;
#1954=EDGE_CURVE ( 'NONE', #7681, #7154, #8463, .T. ) ;
#1955=AXIS2_PLACEMENT_3D ( 'NONE', #6201, #251, #200 ) ;
#1957=CYLINDRICAL_SURFACE ( 'NONE', #5118, 2.500000000000002220 ) ;
#1961=CARTESIAN_POINT ( 'NONE',  ( 4.898587196589413815E-15, 0.000000000000000000, 40.00000000000000711 ) ) ;
#1968=VECTOR ( 'NONE', #9277, 1000.000000000000000 ) ;
#1970=CARTESIAN_POINT ( 'NONE',  ( 16.70299909897254409, 61.99999999999999289, -30.18708036726510002 ) ) ;
#1983=EDGE_LOOP ( 'NONE', ( #9554, #3770, #3275, #7476, #80 ) ) ;
#1986=ORIENTED_EDGE ( 'NONE', *, *, #3474, .F. ) ;
#1994=ORIENTED_EDGE ( 'NONE', *, *, #7366, .F. ) ;
#1995=CARTESIAN_POINT ( 'NONE',  ( -15.97678174684350871, 60.99999999999999289, 28.87459861216650836 ) ) ;
#1998=DIRECTION ( 'NONE',  ( 0.000000000000000000, 1.000000000000000000, 0.000000000000000000 ) ) ;
#1999=CARTESIAN_POINT ( 'NONE',  ( -33.06426808735054124, 69.99999999999998579, -5.562309845534581854 ) ) ;
#2000=ADVANCED_FACE ( 'NONE', ( #6264 ), #8547, .T. ) ;
#2014=ORIENTED_EDGE ( 'NONE', *, *, #5120, .T. ) ;
#2015=EDGE_CURVE ( 'NONE', #2652, #7114, #6681, .T. ) ;
#2017=EDGE_CURVE ( 'NONE', #4254, #1750, #5591, .T. ) ;
#2032=CIRCLE ( 'NONE', #7573, 1.500000000000000888 ) ;
#2035=DIRECTION ( 'NONE',  ( -1.000000000000000000, 0.000000000000000000, -3.083952846180987322E-15 ) ) ;
#2040=DIRECTION ( 'NONE',  ( 0.000000000000000000, -1.000000000000000000, 0.000000000000000000 ) ) ;
#2042=DIRECTION ( 'NONE',  ( -0.000000000000000000, -1.000000000000000000, -0.000000000000000000 ) ) ;
#2046=EDGE_LOOP ( 'NONE', ( #4339, #1311, #9651, #3812, #6005 ) ) ;
#2055=FACE_BOUND ( 'NONE', #7598, .T. ) ;
#2064=DIRECTION ( 'NONE',  ( 0.000000000000000000, 0.000000000000000000, 1.000000000000000000 ) ) ;
#2067=EDGE_CURVE ( 'NONE', #6704, #1432, #9068, .T. ) ;
#2069=ORIENTED_EDGE ( 'NONE', *, *, #6780, .F. ) ;
#2071=ADVANCED_FACE ( 'NONE', ( #8094 ), #9621, .T. ) ;
#2072=VERTEX_POINT ( 'NONE', #639 ) ;
#2089=DIRECTION ( 'NONE',  ( 0.000000000000000000, 1.000000000000000000, 0.000000000000000000 ) ) ;
#2097=DIRECTION ( 'NONE',  ( 0.000000000000000000, 0.000000000000000000, 1.000000000000000000 ) ) ;
#2103=DIRECTION ( 'NONE',  ( 0.000000000000000000, 0.000000000000000000, -1.000000000000000000 ) ) ;
#2105=EDGE_LOOP ( 'NONE', ( #4709, #5925, #3468, #1218 ) ) ;
#2110=CARTESIAN_POINT ( 'NONE',  ( 33.06426808735054124, 59.99999999999999289, 3.062309845534584074 ) ) ;
#2115=VECTOR ( 'NONE', #1072, 1000.000000000000000 ) ;
#2122=DIRECTION ( 'NONE',  ( 0.000000000000000000, 1.000000000000000000, 0.000000000000000000 ) ) ;
#2128=DIRECTION ( 'NONE',  ( 0.000000000000000000, 0.000000000000000000, -1.000000000000000000 ) ) ;
#2137=DIRECTION ( 'NONE',  ( 0.000000000000000000, 0.000000000000000000, 1.000000000000000000 ) ) ;
#2138=DIRECTION ( 'NONE',  ( 0.000000000000000000, 0.000000000000000000, 1.000000000000000000 ) ) ;
#2141=VECTOR ( 'NONE', #299, 1000.000000000000000 ) ;
#2145=CARTESIAN_POINT ( 'NONE',  ( -5.562309845534701758, 61.83753588906734677, 37.56426808735052703 ) ) ;
#2153=CARTESIAN_POINT ( 'NONE',  ( 0.000000000000000000, 61.99999999999999289, -37.00000000000000711 ) ) ;
#2165=ORIENTED_EDGE ( 'NONE', *, *, #7583, .T. ) ;
#2169=VERTEX_POINT ( 'NONE', #1236 ) ;
#2173=DIRECTION ( 'NONE',  ( 0.000000000000000000, 1.000000000000000000, 0.000000000000000000 ) ) ;
#2175=PLANE ( 'NONE',  #7256 ) ;
#2199=CARTESIAN_POINT ( 'NONE',  ( -5.562309845534701758, 60.99999999999999289, 37.56426808735052703 ) ) ;
#2210=VERTEX_POINT ( 'NONE', #9035 ) ;
#2226=DIRECTION ( 'NONE',  ( 0.000000000000000000, -0.000000000000000000, 1.000000000000000000 ) ) ;
#2228=ORIENTED_EDGE ( 'NONE', *, *, #9343, .T. ) ;
#2230=CYLINDRICAL_SURFACE ( 'NONE', #9711, 1.500000000000003109 ) ;
#2231=EDGE_CURVE ( 'NONE', #7884, #2072, #5899, .T. ) ;
#2232=DIRECTION ( 'NONE',  ( -1.000000000000000000, 0.000000000000000000, 0.000000000000000000 ) ) ;
#2237=DIRECTION ( 'NONE',  ( -0.000000000000000000, -1.000000000000000000, -0.000000000000000000 ) ) ;
#2240=EDGE_CURVE ( 'NONE', #9175, #8122, #2898, .T. ) ;
#2245=CARTESIAN_POINT ( 'NONE',  ( 34.07933880998927378, 61.99999999999999289, -5.371095444502794081 ) ) ;
#2251=EDGE_CURVE ( 'NONE', #7059, #7114, #6000, .T. ) ;
#2253=CARTESIAN_POINT ( 'NONE',  ( 5.134502662544400131, 61.85904243767787847, -37.56426808735048439 ) ) ;
#2257=PRODUCT_CONTEXT ( 'NONE', #6297, 'mechanical' ) ;
#2261=CIRCLE ( 'NONE', #7323, 31.49999999999999289 ) ;
#2273=CARTESIAN_POINT ( 'NONE',  ( 5.562309845534932684, 60.99999999999999289, -33.06426808735049150 ) ) ;
#2274=EDGE_LOOP ( 'NONE', ( #2478, #1343, #853, #4650 ) ) ;
#2275=AXIS2_PLACEMENT_3D ( 'NONE', #9603, #8765, #2035 ) ;
#2278=TOROIDAL_SURFACE ( 'NONE', #5907, 37.00000000000000711, 1.000000000000000888 ) ;
#2286=AXIS2_PLACEMENT_3D ( 'NONE', #7474, #4416, #2967 ) ;
#2292=DIRECTION ( 'NONE',  ( 0.000000000000000000, 0.000000000000000000, 1.000000000000000000 ) ) ;
#2293=LINE ( 'NONE', #6833, #1351 ) ;
#2294=VECTOR ( 'NONE', #5837, 1000.000000000000000 ) ;
#2297=PLANE ( 'NONE',  #1122 ) ;
#2308=CYLINDRICAL_SURFACE ( 'NONE', #9506, 1.500000000000001332 ) ;
#2332=CYLINDRICAL_SURFACE ( 'NONE', #2582, 4.500000000000003553 ) ;
#2354=ORIENTED_EDGE ( 'NONE', *, *, #5037, .T. ) ;
#2355=CARTESIAN_POINT ( 'NONE',  ( 5.562309845534588959, 59.99999999999999289, -33.06426808735054124 ) ) ;
#2360=DIRECTION ( 'NONE',  ( -0.000000000000000000, 1.000000000000000000, -0.000000000000000000 ) ) ;
#2382=CARTESIAN_POINT ( 'NONE',  ( 16.70299909897254409, 60.99999999999999289, -30.18708036726510002 ) ) ;
#2384=EDGE_CURVE ( 'NONE', #7811, #3246, #2890, .T. ) ;
#2393=DIRECTION ( 'NONE',  ( 0.000000000000000000, 1.000000000000000000, 0.000000000000000000 ) ) ;
#2394=DIRECTION ( 'NONE',  ( 0.000000000000000000, 0.000000000000000000, -1.000000000000000000 ) ) ;
#2400=ORIENTED_EDGE ( 'NONE', *, *, #41, .T. ) ;
#2405=VERTEX_POINT ( 'NONE', #3903 ) ;
#2407=DIRECTION ( 'NONE',  ( 0.000000000000000000, -1.000000000000000000, 0.000000000000000000 ) ) ;
#2410=DIRECTION ( 'NONE',  ( 0.000000000000000000, 0.000000000000000000, 1.000000000000000000 ) ) ;
#2417=CIRCLE ( 'NONE', #7954, 2.500000000000002220 ) ;
#2419=CIRCLE ( 'NONE', #76, 1.500000000000001332 ) ;
#2424=EDGE_CURVE ( 'NONE', #5694, #2645, #6300, .T. ) ;
#2430=DIRECTION ( 'NONE',  ( 0.000000000000000000, 0.000000000000000000, 1.000000000000000000 ) ) ;
#2432=DIRECTION ( 'NONE',  ( -0.000000000000000000, 1.000000000000000000, -0.000000000000000000 ) ) ;
#2433=FACE_OUTER_BOUND ( 'NONE', #5913, .T. ) ;
#2445=DIRECTION ( 'NONE',  ( 0.000000000000000000, -1.000000000000000000, 0.000000000000000000 ) ) ;
#2446=AXIS2_PLACEMENT_3D ( 'NONE', #272, #3261, #9298 ) ;
#2454=CARTESIAN_POINT ( 'NONE',  ( -5.562309845534584518, 59.99999999999999289, 30.56426808735054124 ) ) ;
#2458=CARTESIAN_POINT ( 'NONE',  ( 4.716066576642940156, 61.89689025924450050, -37.50432491070253604 ) ) ;
#2461=DIRECTION ( 'NONE',  ( 0.000000000000000000, 1.000000000000000000, 0.000000000000000000 ) ) ;
#2465=ORIENTED_EDGE ( 'NONE', *, *, #3112, .T. ) ;
#2468=ORIENTED_EDGE ( 'NONE', *, *, #2534, .T. ) ;
#2473=ORIENTED_EDGE ( 'NONE', *, *, #5704, .F. ) ;
#2477=EDGE_CURVE ( 'NONE', #8414, #903, #7792, .T. ) ;
#2478=ORIENTED_EDGE ( 'NONE', *, *, #411, .T. ) ;
#2481=DIRECTION ( 'NONE',  ( 0.000000000000000000, 0.000000000000000000, 1.000000000000000000 ) ) ;
#2484=FACE_OUTER_BOUND ( 'NONE', #9071, .T. ) ;
#2492=CARTESIAN_POINT ( 'NONE',  ( 8.106025752690735331, 61.92736406916336733, -36.79170325027448030 ) ) ;
#2495=DIRECTION ( 'NONE',  ( 0.000000000000000000, 1.000000000000000000, 0.000000000000000000 ) ) ;
#2496=DIRECTION ( 'NONE',  ( 0.000000000000000000, 0.000000000000000000, 1.000000000000000000 ) ) ;
#2500=EDGE_CURVE ( 'NONE', #344, #2516, #1129, .T. ) ;
#2502=ORIENTED_EDGE ( 'NONE', *, *, #6659, .T. ) ;
#2506=ORIENTED_EDGE ( 'NONE', *, *, #749, .T. ) ;
#2516=VERTEX_POINT ( 'NONE', #4195 ) ;
#2519=EDGE_CURVE ( 'NONE', #8611, #9175, #2419, .T. ) ;
#2521=AXIS2_PLACEMENT_3D ( 'NONE', #331, #2531, #2394 ) ;
#2522=CYLINDRICAL_SURFACE ( 'NONE', #7780, 2.500000000000002220 ) ;
#2531=DIRECTION ( 'NONE',  ( -0.000000000000000000, -1.000000000000000000, -0.000000000000000000 ) ) ;
#2532=LINE ( 'NONE', #5564, #1274 ) ;
#2534=EDGE_CURVE ( 'NONE', #8621, #344, #4179, .T. ) ;
#2541=CARTESIAN_POINT ( 'NONE',  ( 9.082100980773736509, 61.99999999999999289, -35.86802812777734317 ) ) ;
#2553=AXIS2_PLACEMENT_3D ( 'NONE', #4598, #740, #5334 ) ;
#2554=ADVANCED_FACE ( 'NONE', ( #3444 ), #1957, .F. ) ;
#2558=B_SPLINE_CURVE_WITH_KNOTS ( 'NONE', 3,
 ( #2541, #8495, #1862, #2492, #8535, #9284, #8584, #6256, #4881, #392 ),
 .UNSPECIFIED., .F., .F.,
 ( 4, 2, 2, 2, 4 ),
 ( 0.003057178249550609149, 0.004067793317122886214, 0.005078408384695163279, 0.006089023452267437742, 0.007099638519839713072 ),
 .UNSPECIFIED. ) ;
#2561=ADVANCED_FACE ( 'NONE', ( #9258 ), #5275, .F. ) ;
#2574=AXIS2_PLACEMENT_3D ( 'NONE', #8035, #2745, #3488 ) ;
#2577=ORIENTED_EDGE ( 'NONE', *, *, #4692, .F. ) ;
#2581=CARTESIAN_POINT ( 'NONE',  ( 27.56211685706808723, 60.99999999999999289, 15.25056439471416780 ) ) ;
#2582=AXIS2_PLACEMENT_3D ( 'NONE', #4626, #6968, #3774 ) ;
#2584=AXIS2_PLACEMENT_3D ( 'NONE', #6507, #455, #7302 ) ;
#2591=CARTESIAN_POINT ( 'NONE',  ( 33.06426808735054124, 61.99999999999999289, 5.562309845534586294 ) ) ;
#2596=DIRECTION ( 'NONE',  ( 0.000000000000000000, -1.000000000000000000, 0.000000000000000000 ) ) ;
#2598=CIRCLE ( 'NONE', #2762, 37.00000000000000711 ) ;
#2601=EDGE_CURVE ( 'NONE', #4748, #341, #8273, .T. ) ;
#2604=CIRCLE ( 'NONE', #3077, 34.50000000000000000 ) ;
#2605=VECTOR ( 'NONE', #2360, 1000.000000000000000 ) ;
#2617=EDGE_CURVE ( 'NONE', #7114, #5836, #4018, .T. ) ;
#2620=CARTESIAN_POINT ( 'NONE',  ( 5.562309845534932684, 60.99999999999999289, -28.56426808735048439 ) ) ;
#2626=ORIENTED_EDGE ( 'NONE', *, *, #4565, .F. ) ;
#2629=DIRECTION ( 'NONE',  ( 0.000000000000000000, 0.000000000000000000, 1.000000000000000000 ) ) ;
#2631=ORIENTED_EDGE ( 'NONE', *, *, #6119, .F. ) ;
#2645=VERTEX_POINT ( 'NONE', #3032 ) ;
#2649=CARTESIAN_POINT ( 'NONE',  ( -37.38678512219217254, 61.82631808411006347, -6.843790051325325585 ) ) ;
#2652=VERTEX_POINT ( 'NONE', #7548 ) ;
#2655=EDGE_LOOP ( 'NONE', ( #7603, #2961, #1699, #297 ) ) ;
#2656=CYLINDRICAL_SURFACE ( 'NONE', #6642, 2.500000000000002220 ) ;
#2660=( NAMED_UNIT ( * ) SI_UNIT ( $, .STERADIAN. ) SOLID_ANGLE_UNIT ( ) );
#2661=ADVANCED_FACE ( 'NONE', ( #5176 ), #1198, .T. ) ;
#2668=ORIENTED_EDGE ( 'NONE', *, *, #5762, .T. ) ;
#2670=EDGE_CURVE ( 'NONE', #4372, #4366, #4200, .T. ) ;
#2671=CARTESIAN_POINT ( 'NONE',  ( 4.904043666719842598, 60.99999999999999289, 31.11591804390326743 ) ) ;
#2675=CIRCLE ( 'NONE', #5532, 31.50000000000000000 ) ;
#2683=CARTESIAN_POINT ( 'NONE',  ( -33.06426808735054124, 59.99999999999999289, -3.062309845534580077 ) ) ;
#2688=EDGE_CURVE ( 'NONE', #1639, #7141, #7341, .T. ) ;
#2692=DIRECTION ( 'NONE',  ( 0.000000000000000000, 0.000000000000000000, -1.000000000000000000 ) ) ;
#2694=CARTESIAN_POINT ( 'NONE',  ( 33.06426808735054124, 61.99999999999999289, 5.562309845534586294 ) ) ;
#2695=( NAMED_UNIT ( * ) SI_UNIT ( $, .STERADIAN. ) SOLID_ANGLE_UNIT ( ) );
#2698=DIRECTION ( 'NONE',  ( -0.000000000000000000, -1.000000000000000000, -0.000000000000000000 ) ) ;
#2699=CIRCLE ( 'NONE', #4140, 1.499999999999999556 ) ;
#2715=CARTESIAN_POINT ( 'NONE',  ( -33.06426808735054124, 59.99999999999999289, -5.562309845534581854 ) ) ;
#2719=VERTEX_POINT ( 'NONE', #1412 ) ;
#2723=EDGE_CURVE ( 'NONE', #9614, #3486, #2293, .T. ) ;
#2727=DIRECTION ( 'NONE',  ( -0.000000000000000000, -1.000000000000000000, -0.000000000000000000 ) ) ;
#2737=DIRECTION ( 'NONE',  ( 0.000000000000000000, 0.000000000000000000, -1.000000000000000000 ) ) ;
#2739=ADVANCED_FACE ( 'NONE', ( #8710 ), #7016, .F. ) ;
#2744=DIRECTION ( 'NONE',  ( 0.000000000000000000, 0.000000000000000000, 1.000000000000000000 ) ) ;
#2745=DIRECTION ( 'NONE',  ( 0.000000000000000000, 1.000000000000000000, 0.000000000000000000 ) ) ;
#2749=( LENGTH_UNIT ( ) NAMED_UNIT ( * ) SI_UNIT ( .MILLI., .METRE. ) );
#2752=CIRCLE ( 'NONE', #5454, 1.500000000000001332 ) ;
#2756=ORIENTED_EDGE ( 'NONE', *, *, #3040, .F. ) ;
#2762=AXIS2_PLACEMENT_3D ( 'NONE', #3215, #3317, #957 ) ;
#2770=FACE_OUTER_BOUND ( 'NONE', #4251, .T. ) ;
#2773=LINE ( 'NONE', #5792, #6923 ) ;
#2778=CYLINDRICAL_SURFACE ( 'NONE', #727, 2.500000000000001332 ) ;
#2783=DIRECTION ( 'NONE',  ( 0.000000000000000000, 1.000000000000000000, 0.000000000000000000 ) ) ;
#2799=ADVANCED_FACE ( 'NONE', ( #7875 ), #6377, .F. ) ;
#2802=DIRECTION ( 'NONE',  ( 0.000000000000000000, 0.000000000000000000, 1.000000000000000000 ) ) ;
#2812=DIRECTION ( 'NONE',  ( 0.000000000000000000, 1.000000000000000000, 0.000000000000000000 ) ) ;
#2813=AXIS2_PLACEMENT_3D ( 'NONE', #1995, #2783, #4281 ) ;
#2826=ORIENTED_EDGE ( 'NONE', *, *, #4692, .T. ) ;
#2830=DIRECTION ( 'NONE',  ( 0.000000000000000000, 0.000000000000000000, 1.000000000000000000 ) ) ;
#2831=CYLINDRICAL_SURFACE ( 'NONE', #3963, 31.50000000000000000 ) ;
#2837=CARTESIAN_POINT ( 'NONE',  ( 0.000000000000000000, 60.99999999999999289, 0.000000000000000000 ) ) ;
#2853=AXIS2_PLACEMENT_3D ( 'NONE', #6562, #9585, #2802 ) ;
#2855=FACE_OUTER_BOUND ( 'NONE', #3763, .T. ) ;
#2856=CARTESIAN_POINT ( 'NONE',  ( 0.000000000000000000, 60.99999999999999289, 0.000000000000000000 ) ) ;
#2867=LINE ( 'NONE', #1067, #2294 ) ;
#2870=CARTESIAN_POINT ( 'NONE',  ( 0.000000000000000000, 61.99999999999999289, 0.000000000000000000 ) ) ;
#2886=CARTESIAN_POINT ( 'NONE',  ( 0.000000000000000000, 58.99999999999999289, 0.000000000000000000 ) ) ;
#2890=CIRCLE ( 'NONE', #7317, 4.500000000000004441 ) ;
#2898=CIRCLE ( 'NONE', #4187, 31.50000000000000000 ) ;
#2902=ORIENTED_EDGE ( 'NONE', *, *, #9158, .T. ) ;
#2904=CIRCLE ( 'NONE', #3706, 4.500000000000005329 ) ;
#2928=SHAPE_REPRESENTATION ( 'Covrt plate', ( #6314 ), #3968 ) ;
#2929=CIRCLE ( 'NONE', #6867, 4.500000000000005329 ) ;
#2932=ORIENTED_EDGE ( 'NONE', *, *, #350, .F. ) ;
#2940=DIRECTION ( 'NONE',  ( -0.000000000000000000, -1.000000000000000000, -0.000000000000000000 ) ) ;
#2941=DIRECTION ( 'NONE',  ( 0.000000000000000000, 0.000000000000000000, 1.000000000000000000 ) ) ;
#2953=DIRECTION ( 'NONE',  ( 0.000000000000000000, 0.000000000000000000, -1.000000000000000000 ) ) ;
#2961=ORIENTED_EDGE ( 'NONE', *, *, #9244, .T. ) ;
#2962=FACE_OUTER_BOUND ( 'NONE', #1781, .T. ) ;
#2967=DIRECTION ( 'NONE',  ( 0.000000000000000000, 0.000000000000000000, -1.000000000000000000 ) ) ;
#2985=DIRECTION ( 'NONE',  ( 0.000000000000000000, 0.000000000000000000, 1.000000000000000000 ) ) ;
#2999=DIRECTION ( 'NONE',  ( 0.000000000000000000, 1.000000000000000000, 0.000000000000000000 ) ) ;
#3000=CARTESIAN_POINT ( 'NONE',  ( 3.153634179030674556, 61.99999999999999289, -36.86535760663186068 ) ) ;
#3001=ADVANCED_FACE ( 'NONE', ( #2962 ), #2278, .F. ) ;
#3014=CARTESIAN_POINT ( 'NONE',  ( -3.153634179030417872, 61.99999999999999289, 36.86535760663188199 ) ) ;
#3016=ORIENTED_EDGE ( 'NONE', *, *, #889, .T. ) ;
#3032=CARTESIAN_POINT ( 'NONE',  ( -5.371095444502437921, 61.99999999999999289, -34.07933880998933773 ) ) ;
#3040=EDGE_CURVE ( 'NONE', #7361, #3246, #8255, .T. ) ;
#3048=CARTESIAN_POINT ( 'NONE',  ( 4.104483837744082209, 61.95009619975343185, -37.32687308866057663 ) ) ;
#3055=CIRCLE ( 'NONE', #5745, 1.000000000000000888 ) ;
#3057=ORIENTED_EDGE ( 'NONE', *, *, #9280, .T. ) ;
#3077=AXIS2_PLACEMENT_3D ( 'NONE', #4002, #5492, #2496 ) ;
#3088=CARTESIAN_POINT ( 'NONE',  ( 15.25056439471407188, 61.99999999999999289, -27.56211685706813341 ) ) ;
#3094=ORIENTED_EDGE ( 'NONE', *, *, #1386, .F. ) ;
#3106=CYLINDRICAL_SURFACE ( 'NONE', #7673, 1.500000000000000888 ) ;
#3112=EDGE_CURVE ( 'NONE', #8252, #7059, #8916, .T. ) ;
#3115=CARTESIAN_POINT ( 'NONE',  ( 32.59762842694625817, 60.99999999999999289, -3.637569555611369854 ) ) ;
#3116=CARTESIAN_POINT ( 'NONE',  ( -4.716066576642697683, 61.89689025924450760, 37.50432491070257868 ) ) ;
#3124=EDGE_CURVE ( 'NONE', #7306, #8835, #6688, .T. ) ;
#3141=DIRECTION ( 'NONE',  ( -1.000000000000000000, 0.000000000000000000, -3.083952846180987322E-15 ) ) ;
#3144=CARTESIAN_POINT ( 'NONE',  ( 37.13646476935431195, 61.98650506287648909, 3.627735144839754344 ) ) ;
#3147=DIRECTION ( 'NONE',  ( 0.000000000000000000, 0.000000000000000000, 1.000000000000000000 ) ) ;
#3158=ORIENTED_EDGE ( 'NONE', *, *, #7254, .T. ) ;
#3159=CARTESIAN_POINT ( 'NONE',  ( -30.18708036726492594, 60.99999999999999289, -16.70299909897287094 ) ) ;
#3161=ORIENTED_EDGE ( 'NONE', *, *, #5301, .T. ) ;
#3163=CARTESIAN_POINT ( 'NONE',  ( 0.000000000000000000, 60.99999999999999289, 0.000000000000000000 ) ) ;
#3171=ORIENTED_EDGE ( 'NONE', *, *, #3652, .F. ) ;
#3172=FACE_OUTER_BOUND ( 'NONE', #9211, .T. ) ;
#3176=ORIENTED_EDGE ( 'NONE', *, *, #2251, .F. ) ;
#3183=DIRECTION ( 'NONE',  ( 0.000000000000000000, -1.000000000000000000, 0.000000000000000000 ) ) ;
#3188=CARTESIAN_POINT ( 'NONE',  ( -33.06426808735054124, 60.99999999999999289, -5.562309845534586294 ) ) ;
#3190=AXIS2_PLACEMENT_3D ( 'NONE', #7298, #6557, #2430 ) ;
#3193=CARTESIAN_POINT ( 'NONE',  ( -5.371095444502437921, 60.99999999999999289, -34.07933880998933773 ) ) ;
#3205=DIRECTION ( 'NONE',  ( -0.000000000000000000, -1.000000000000000000, -0.000000000000000000 ) ) ;
#3209=B_SPLINE_CURVE_WITH_KNOTS ( 'NONE', 3,
 ( #3605, #2253, #2458, #3048, #4605, #6853, #9240, #3000 ),
 .UNSPECIFIED., .F., .F.,
 ( 4, 2, 2, 4 ),
 ( 0.007099638519839713072, 0.008372149287075639906, 0.009008404670693602456, 0.009644660054311566741 ),
 .UNSPECIFIED. ) ;
#3212=VECTOR ( 'NONE', #390, 1000.000000000000000 ) ;
#3214=ORIENTED_EDGE ( 'NONE', *, *, #1947, .F. ) ;
#3215=CARTESIAN_POINT ( 'NONE',  ( 0.000000000000000000, 59.99999999999999289, 0.000000000000000000 ) ) ;
#3221=ADVANCED_FACE ( 'NONE', ( #3305 ), #9292, .F. ) ;
#3224=CARTESIAN_POINT ( 'NONE',  ( 31.11591804390324612, 60.99999999999999289, -4.904043666719942074 ) ) ;
#3238=AXIS2_PLACEMENT_3D ( 'NONE', #8197, #7460, #8946 ) ;
#3246=VERTEX_POINT ( 'NONE', #4802 ) ;
#3247=DIRECTION ( 'NONE',  ( 0.000000000000000000, 1.000000000000000000, 0.000000000000000000 ) ) ;
#3254=ORIENTED_EDGE ( 'NONE', *, *, #3417, .F. ) ;
#3261=DIRECTION ( 'NONE',  ( 0.000000000000000000, 1.000000000000000000, 0.000000000000000000 ) ) ;
#3263=CYLINDRICAL_SURFACE ( 'NONE', #9553, 4.500000000000005329 ) ;
#3275=ORIENTED_EDGE ( 'NONE', *, *, #2500, .T. ) ;
#3278=DIRECTION ( 'NONE',  ( -0.000000000000000000, 1.000000000000000000, -0.000000000000000000 ) ) ;
#3282=EDGE_CURVE ( 'NONE', #1736, #5322, #3872, .T. ) ;
#3285=ADVANCED_FACE ( 'NONE', ( #5035, #502, #5727, #9482, #1191, #8743 ), #5140, .T. ) ;
#3292=ORIENTED_EDGE ( 'NONE', *, *, #526, .F. ) ;
#3293=CARTESIAN_POINT ( 'NONE',  ( 5.137569555611264605, 60.99999999999999289, 34.09762842694627949 ) ) ;
#3301=CARTESIAN_POINT ( 'NONE',  ( -31.11591804390328164, 60.99999999999999289, 4.904043666719710259 ) ) ;
#3305=FACE_OUTER_BOUND ( 'NONE', #617, .T. ) ;
#3306=EDGE_LOOP ( 'NONE', ( #3395, #5458, #8504, #6267 ) ) ;
#3309=AXIS2_PLACEMENT_3D ( 'NONE', #1163, #7180, #1216 ) ;
#3314=PRODUCT_DEFINITION_CONTEXT ( 'detailed design', #6802, 'design' ) ;
#3315=AXIS2_PLACEMENT_3D ( 'NONE', #5169, #2089, #2138 ) ;
#3317=DIRECTION ( 'NONE',  ( -0.000000000000000000, -1.000000000000000000, -0.000000000000000000 ) ) ;
#3329=CIRCLE ( 'NONE', #8859, 1.000000000000000888 ) ;
#3332=EDGE_CURVE ( 'NONE', #3433, #2169, #2904, .T. ) ;
#3333=CARTESIAN_POINT ( 'NONE',  ( -33.06426808735054124, 60.99999999999999289, -5.562309845534581854 ) ) ;
#3340=VERTEX_POINT ( 'NONE', #1970 ) ;
#3341=CARTESIAN_POINT ( 'NONE',  ( 5.137569555611264605, 60.99999999999999289, 34.09762842694627949 ) ) ;
#3353=CARTESIAN_POINT ( 'NONE',  ( -37.34143203299149860, 61.94837758590841759, -4.137096292553819055 ) ) ;
#3360=CARTESIAN_POINT ( 'NONE',  ( 27.56211685706808723, 61.99999999999999289, 15.25056439471416780 ) ) ;
#3363=DIRECTION ( 'NONE',  ( 0.000000000000000000, 1.000000000000000000, 0.000000000000000000 ) ) ;
#3373=CARTESIAN_POINT ( 'NONE',  ( 15.97678174684330799, 60.99999999999999289, -28.87459861216662205 ) ) ;
#3374=DIRECTION ( 'NONE',  ( 0.000000000000000000, 0.000000000000000000, -1.000000000000000000 ) ) ;
#3376=ORIENTED_EDGE ( 'NONE', *, *, #3649, .F. ) ;
#3378=EDGE_CURVE ( 'NONE', #1432, #3849, #1239, .T. ) ;
#3379=ORIENTED_EDGE ( 'NONE', *, *, #8103, .T. ) ;
#3390=DIRECTION ( 'NONE',  ( -0.000000000000000000, -1.000000000000000000, -0.000000000000000000 ) ) ;
#3391=ORIENTED_EDGE ( 'NONE', *, *, #3648, .F. ) ;
#3395=ORIENTED_EDGE ( 'NONE', *, *, #5657, .F. ) ;
#3397=CARTESIAN_POINT ( 'NONE',  ( -5.562309845534584518, 60.99999999999999289, 33.06426808735054124 ) ) ;
#3400=DIRECTION ( 'NONE',  ( 1.000000000000000000, 0.000000000000000000, -1.224646799147353207E-16 ) ) ;
#3401=AXIS2_PLACEMENT_3D ( 'NONE', #7555, #9134, #6794 ) ;
#3405=CARTESIAN_POINT ( 'NONE',  ( -37.13646476935431195, 61.98650506287648909, -3.627735144839754344 ) ) ;
#3406=AXIS2_PLACEMENT_3D ( 'NONE', #3986, #3278, #6978 ) ;
#3408=FACE_OUTER_BOUND ( 'NONE', #4399, .T. ) ;
#3413=DIRECTION ( 'NONE',  ( 0.000000000000000000, 0.000000000000000000, 1.000000000000000000 ) ) ;
#3416=STYLED_ITEM('',(#9785),#9444);
#3417=EDGE_CURVE ( 'NONE', #4234, #9299, #4786, .T. ) ;
#3433=VERTEX_POINT ( 'NONE', #6109 ) ;
#3437=DIRECTION ( 'NONE',  ( -0.000000000000000000, -1.000000000000000000, -0.000000000000000000 ) ) ;
#3440=DIRECTION ( 'NONE',  ( -0.000000000000000000, -1.000000000000000000, -0.000000000000000000 ) ) ;
#3442=ORIENTED_EDGE ( 'NONE', *, *, #9410, .T. ) ;
#3444=FACE_OUTER_BOUND ( 'NONE', #3489, .T. ) ;
#3451=DIRECTION ( 'NONE',  ( -0.000000000000000000, 1.000000000000000000, -0.000000000000000000 ) ) ;
#3460=ADVANCED_FACE ( 'NONE', ( #8192 ), #9187, .F. ) ;
#3463=SHAPE_REPRESENTATION_RELATIONSHIP ( 'NONE' , 'NONE' ,  #2928, #6901 ) ;
#3467=CARTESIAN_POINT ( 'NONE',  ( 0.000000000000000000, 0.000000000000000000, 0.000000000000000000 ) ) ;
#3468=ORIENTED_EDGE ( 'NONE', *, *, #1126, .F. ) ;
#3471=FACE_OUTER_BOUND ( 'NONE', #6494, .T. ) ;
#3474=EDGE_CURVE ( 'NONE', #341, #4748, #1938, .T. ) ;
#3486=VERTEX_POINT ( 'NONE', #2245 ) ;
#3488=DIRECTION ( 'NONE',  ( 1.000000000000000000, 0.000000000000000000, 1.079383496163345602E-14 ) ) ;
#3489=EDGE_LOOP ( 'NONE', ( #4662, #4209, #1880, #3254 ) ) ;
#3492=CARTESIAN_POINT ( 'NONE',  ( 4.653657836759942730E-15, 58.99999999999999289, 38.00000000000000711 ) ) ;
#3496=B_SPLINE_CURVE_WITH_KNOTS ( 'NONE', 3,
 ( #5527, #7702, #9235, #8496, #1720, #7652, #9374, #934, #3906, #4741, #981, #9285, #6894, #6942, #155, #3144, #6158, #7746 ),
 .UNSPECIFIED., .F., .F.,
 ( 4, 2, 2, 2, 2, 2, 2, 2, 4 ),
 ( 0.003057178249550605680, 0.003880613475145725487, 0.004704048700740845294, 0.005527483926335964234, 0.006350919151931084042, 0.007174354377526204717, 0.007997789603121323657, 0.008821224828716443464, 0.009644660054311565006 ),
 .UNSPECIFIED. ) ;
#3497=CARTESIAN_POINT ( 'NONE',  ( -15.97678174684350871, 61.99999999999999289, 28.87459861216650836 ) ) ;
#3498=VERTEX_POINT ( 'NONE', #8342 ) ;
#3509=ORIENTED_EDGE ( 'NONE', *, *, #1126, .T. ) ;
#3520=DIRECTION ( 'NONE',  ( 0.000000000000000000, 0.000000000000000000, 1.000000000000000000 ) ) ;
#3534=CARTESIAN_POINT ( 'NONE',  ( 0.000000000000000000, 60.99999999999999289, 0.000000000000000000 ) ) ;
#3535=VECTOR ( 'NONE', #6356, 1000.000000000000000 ) ;
#3537=AXIS2_PLACEMENT_3D ( 'NONE', #3497, #4298, #499 ) ;
#3540=EDGE_CURVE ( 'NONE', #8683, #5164, #845, .T. ) ;
#3549=CIRCLE ( 'NONE', #5288, 2.500000000000002220 ) ;
#3561=DIRECTION ( 'NONE',  ( 0.000000000000000000, 1.000000000000000000, 0.000000000000000000 ) ) ;
#3575=CARTESIAN_POINT ( 'NONE',  ( 4.898587196589413815E-15, 52.29648987751954792, 40.00000000000000711 ) ) ;
#3576=VECTOR ( 'NONE', #8552, 1000.000000000000000 ) ;
#3581=CARTESIAN_POINT ( 'NONE',  ( -33.06426808735054124, 61.99999999999999289, -1.062309845534581632 ) ) ;
#3583=DIRECTION ( 'NONE',  ( -0.000000000000000000, 1.000000000000000000, -0.000000000000000000 ) ) ;
#3586=EDGE_CURVE ( 'NONE', #1101, #6057, #9090, .T. ) ;
#3587=DIRECTION ( 'NONE',  ( -0.000000000000000000, -1.000000000000000000, -0.000000000000000000 ) ) ;
#3593=DIRECTION ( 'NONE',  ( 0.000000000000000000, 0.000000000000000000, 1.000000000000000000 ) ) ;
#3600=EDGE_LOOP ( 'NONE', ( #9251, #3738, #281, #1341 ) ) ;
#3605=CARTESIAN_POINT ( 'NONE',  ( 5.562309845534932684, 61.83753588906734677, -37.56426808735049150 ) ) ;
#3609=ORIENTED_EDGE ( 'NONE', *, *, #1241, .F. ) ;
#3614=DIRECTION ( 'NONE',  ( 0.000000000000000000, 0.000000000000000000, -1.000000000000000000 ) ) ;
#3619=AXIS2_PLACEMENT_3D ( 'NONE', #1705, #4723, #3831 ) ;
#3639=CARTESIAN_POINT ( 'NONE',  ( 5.562309845534588959, 59.99999999999999289, -30.56426808735054479 ) ) ;
#3642=DIRECTION ( 'NONE',  ( 0.000000000000000000, 0.000000000000000000, -1.000000000000000000 ) ) ;
#3644=EDGE_LOOP ( 'NONE', ( #9144, #2354, #6872, #7522 ) ) ;
#3648=EDGE_CURVE ( 'NONE', #7858, #1498, #7701, .T. ) ;
#3649=EDGE_CURVE ( 'NONE', #8122, #6057, #1628, .T. ) ;
#3650=EDGE_CURVE ( 'NONE', #4765, #5790, #2558, .T. ) ;
#3652=EDGE_CURVE ( 'NONE', #7154, #9614, #222, .T. ) ;
#3656=ORIENTED_EDGE ( 'NONE', *, *, #6659, .F. ) ;
#3660=ORIENTED_EDGE ( 'NONE', *, *, #9410, .F. ) ;
#3664=ORIENTED_EDGE ( 'NONE', *, *, #4032, .F. ) ;
#3674=AXIS2_PLACEMENT_3D ( 'NONE', #8021, #9458, #476 ) ;
#3683=DIRECTION ( 'NONE',  ( -0.000000000000000000, 1.000000000000000000, -0.000000000000000000 ) ) ;
#3685=DIRECTION ( 'NONE',  ( 0.000000000000000000, 0.000000000000000000, -1.000000000000000000 ) ) ;
#3691=AXIS2_PLACEMENT_3D ( 'NONE', #241, #6244, #8865 ) ;
#3695=ORIENTED_EDGE ( 'NONE', *, *, #6944, .F. ) ;
#3699=AXIS2_PLACEMENT_3D ( 'NONE', #5575, #6021, #5972 ) ;
#3706=AXIS2_PLACEMENT_3D ( 'NONE', #7304, #5864, #457 ) ;
#3707=ADVANCED_FACE ( 'NONE', ( #4699, #7745 ), #8640, .T. ) ;
#3712=EDGE_CURVE ( 'NONE', #7580, #5699, #56, .T. ) ;
#3735=DIRECTION ( 'NONE',  ( 0.000000000000000000, 0.000000000000000000, 1.000000000000000000 ) ) ;
#3738=ORIENTED_EDGE ( 'NONE', *, *, #8889, .F. ) ;
#3743=AXIS2_PLACEMENT_3D ( 'NONE', #2837, #447, #2744 ) ;
#3763=EDGE_LOOP ( 'NONE', ( #459, #8108, #6903, #3974, #5360 ) ) ;
#3764=FACE_OUTER_BOUND ( 'NONE', #5628, .T. ) ;
#3765=EDGE_CURVE ( 'NONE', #7319, #7328, #9668, .T. ) ;
#3766=CARTESIAN_POINT ( 'NONE',  ( -2.568784777805515507, 60.99999999999999289, -16.29881421347316106 ) ) ;
#3768=ORIENTED_EDGE ( 'NONE', *, *, #2015, .T. ) ;
#3770=ORIENTED_EDGE ( 'NONE', *, *, #8179, .F. ) ;
#3774=DIRECTION ( 'NONE',  ( 0.000000000000000000, 0.000000000000000000, 1.000000000000000000 ) ) ;
#3779=DIRECTION ( 'NONE',  ( -0.000000000000000000, -1.000000000000000000, -0.000000000000000000 ) ) ;
#3785=CARTESIAN_POINT ( 'NONE',  ( -6.890850105526180158, 61.82663791069490600, 37.37679511928145359 ) ) ;
#3787=DIRECTION ( 'NONE',  ( -0.000000000000000000, -1.000000000000000000, -0.000000000000000000 ) ) ;
#3797=DIRECTION ( 'NONE',  ( -0.000000000000000000, 1.000000000000000000, -0.000000000000000000 ) ) ;
#3798=ORIENTED_EDGE ( 'NONE', *, *, #8889, .T. ) ;
#3799=CARTESIAN_POINT ( 'NONE',  ( 0.000000000000000000, 58.99999999999999289, 0.000000000000000000 ) ) ;
#3803=DIRECTION ( 'NONE',  ( -0.000000000000000000, 1.000000000000000000, -0.000000000000000000 ) ) ;
#3812=ORIENTED_EDGE ( 'NONE', *, *, #480, .T. ) ;
#3813=DIRECTION ( 'NONE',  ( 0.000000000000000000, 0.000000000000000000, 1.000000000000000000 ) ) ;
#3816=CARTESIAN_POINT ( 'NONE',  ( 0.000000000000000000, 0.000000000000000000, -27.99999999999999289 ) ) ;
#3831=DIRECTION ( 'NONE',  ( 1.000000000000000000, 0.000000000000000000, 1.047444401652940007E-14 ) ) ;
#3832=AXIS2_PLACEMENT_3D ( 'NONE', #3996, #4148, #1678 ) ;
#3839=CYLINDRICAL_SURFACE ( 'NONE', #426, 2.500000000000002220 ) ;
#3842=ORIENTED_EDGE ( 'NONE', *, *, #5826, .F. ) ;
#3849=VERTEX_POINT ( 'NONE', #594 ) ;
#3859=DIRECTION ( 'NONE',  ( -0.000000000000000000, 1.000000000000000000, -0.000000000000000000 ) ) ;
#3865=AXIS2_PLACEMENT_3D ( 'NONE', #552, #3451, #6453 ) ;
#3869=CARTESIAN_POINT ( 'NONE',  ( 0.000000000000000000, 52.29648987751954792, 0.000000000000000000 ) ) ;
#3872=CIRCLE ( 'NONE', #8445, 37.00000000000000711 ) ;
#3874=CARTESIAN_POINT ( 'NONE',  ( -4.904043666719616112, 60.99999999999999289, -31.11591804390330651 ) ) ;
#3877=EDGE_LOOP ( 'NONE', ( #8886, #8898 ) ) ;
#3881=CIRCLE ( 'NONE', #1500, 34.49999999999999289 ) ;
#3884=DIRECTION ( 'NONE',  ( -0.000000000000000000, 1.000000000000000000, -0.000000000000000000 ) ) ;
#3888=FACE_OUTER_BOUND ( 'NONE', #8164, .T. ) ;
#3890=ADVANCED_FACE ( 'NONE', ( #5815 ), #8827, .F. ) ;
#3893=CIRCLE ( 'NONE', #9414, 1.500000000000003109 ) ;
#3897=ORIENTED_EDGE ( 'NONE', *, *, #8796, .T. ) ;
#3898=CLOSED_SHELL ( 'NONE', ( #431, #5580, #3890, #1849, #4758, #6419, #5465, #1528, #1934, #3001, #1254, #1509, #9689, #6964, #8787, #7769, #6610, #6038, #2554, #7675, #9746, #8939, #7485, #2661, #3285, #2739, #373, #2561, #2799, #1608, #5281, #1472, #296, #8091, #3707, #5877, #8833, #8548, #8967, #6472, #3221, #8413, #7260, #5355, #5001, #8777, #5048, #6187, #2000, #4808, #510, #4814, #3460, #2071, #1306, #8128, #6772 ) ) ;
#3903=CARTESIAN_POINT ( 'NONE',  ( -9.082100980773482490, 61.99999999999999289, 35.86802812777740002 ) ) ;
#3906=CARTESIAN_POINT ( 'NONE',  ( 37.45692540970868833, 61.81802411364413530, 6.576816292457711377 ) ) ;
#3911=EDGE_CURVE ( 'NONE', #903, #8414, #198, .T. ) ;
#3918=ORIENTED_EDGE ( 'NONE', *, *, #3417, .T. ) ;
#3921=LINE ( 'NONE', #3115, #6556 ) ;
#3945=DIRECTION ( 'NONE',  ( -0.000000000000000000, 1.000000000000000000, -0.000000000000000000 ) ) ;
#3949=LINE ( 'NONE', #4649, #2141 ) ;
#3957=EDGE_CURVE ( 'NONE', #5836, #2719, #2699, .T. ) ;
#3962=LINE ( 'NONE', #216, #8935 ) ;
#3963=AXIS2_PLACEMENT_3D ( 'NONE', #582, #3583, #8919 ) ;
#3968=( GEOMETRIC_REPRESENTATION_CONTEXT ( 3 ) GLOBAL_UNCERTAINTY_ASSIGNED_CONTEXT ( ( #5257 ) ) GLOBAL_UNIT_ASSIGNED_CONTEXT ( ( #7163, #465, #2660 ) ) REPRESENTATION_CONTEXT ( 'NONE', 'WORKASPACE' ) );
#3970=FACE_OUTER_BOUND ( 'NONE', #1002, .T. ) ;
#3973=ORIENTED_EDGE ( 'NONE', *, *, #4862, .T. ) ;
#3974=ORIENTED_EDGE ( 'NONE', *, *, #3124, .T. ) ;
#3982=DIRECTION ( 'NONE',  ( -0.000000000000000000, 1.000000000000000000, -0.000000000000000000 ) ) ;
#3984=DIRECTION ( 'NONE',  ( 0.000000000000000000, 1.000000000000000000, 0.000000000000000000 ) ) ;
#3986=CARTESIAN_POINT ( 'NONE',  ( 0.000000000000000000, 60.99999999999999289, 0.000000000000000000 ) ) ;
#3989=DIRECTION ( 'NONE',  ( 0.000000000000000000, 1.000000000000000000, 0.000000000000000000 ) ) ;
#3996=CARTESIAN_POINT ( 'NONE',  ( 0.000000000000000000, 58.99999999999999289, 0.000000000000000000 ) ) ;
#4002=CARTESIAN_POINT ( 'NONE',  ( 0.000000000000000000, 60.99999999999999289, 0.000000000000000000 ) ) ;
#4006=ORIENTED_EDGE ( 'NONE', *, *, #7402, .T. ) ;
#4008=CARTESIAN_POINT ( 'NONE',  ( -31.11591804390328164, 60.99999999999999289, 4.904043666719710259 ) ) ;
#4018=CIRCLE ( 'NONE', #9534, 31.49999999999999289 ) ;
#4019=EDGE_LOOP ( 'NONE', ( #7516, #7577 ) ) ;
#4021=EDGE_CURVE ( 'NONE', #6202, #9175, #4086, .T. ) ;
#4024=EDGE_LOOP ( 'NONE', ( #5383, #7669, #695, #6241 ) ) ;
#4027=CARTESIAN_POINT ( 'NONE',  ( -5.562309845534701758, 60.99999999999999289, 33.06426808735052703 ) ) ;
#4028=AXIS2_PLACEMENT_3D ( 'NONE', #4530, #2042, #583 ) ;
#4032=EDGE_CURVE ( 'NONE', #7590, #4511, #4924, .T. ) ;
#4041=DIRECTION ( 'NONE',  ( -1.000000000000000000, 0.000000000000000000, -3.083952846180987322E-15 ) ) ;
#4043=VECTOR ( 'NONE', #5830, 1000.000000000000000 ) ;
#4049=CARTESIAN_POINT ( 'NONE',  ( 32.59762842694625817, 60.99999999999999289, -5.137569555611371186 ) ) ;
#4054=DIRECTION ( 'NONE',  ( 0.000000000000000000, 0.000000000000000000, -1.000000000000000000 ) ) ;
#4056=CARTESIAN_POINT ( 'NONE',  ( -36.28089590215267179, 61.98637676474528746, -8.721193672020515208 ) ) ;
#4059=DIRECTION ( 'NONE',  ( -0.000000000000000000, 1.000000000000000000, -0.000000000000000000 ) ) ;
#4061=ORIENTED_EDGE ( 'NONE', *, *, #3540, .F. ) ;
#4081=ORIENTED_EDGE ( 'NONE', *, *, #5215, .T. ) ;
#4086=LINE ( 'NONE', #2581, #512 ) ;
#4089=LINE ( 'NONE', #6344, #5214 ) ;
#4091=CARTESIAN_POINT ( 'NONE',  ( -16.70299909897276081, 60.99999999999999289, 30.18708036726496857 ) ) ;
#4096=CARTESIAN_POINT ( 'NONE',  ( -5.562309845534701758, 61.99999999999999289, 33.06426808735052703 ) ) ;
#4102=CARTESIAN_POINT ( 'NONE',  ( 33.06426808735054124, 61.99999999999999289, 1.062309845534581632 ) ) ;
#4103=CARTESIAN_POINT ( 'NONE',  ( -37.08058572124223673, 61.87769929713620343, -7.610216775991024640 ) ) ;
#4108=DIRECTION ( 'NONE',  ( -0.000000000000000000, -1.000000000000000000, -0.000000000000000000 ) ) ;
#4116=DIRECTION ( 'NONE',  ( 0.000000000000000000, 1.000000000000000000, 0.000000000000000000 ) ) ;
#4120=ORIENTED_EDGE ( 'NONE', *, *, #335, .F. ) ;
#4121=ORIENTED_EDGE ( 'NONE', *, *, #3648, .T. ) ;
#4123=ORIENTED_EDGE ( 'NONE', *, *, #6730, .F. ) ;
#4128=DIRECTION ( 'NONE',  ( 0.000000000000000000, 1.000000000000000000, 0.000000000000000000 ) ) ;
#4140=AXIS2_PLACEMENT_3D ( 'NONE', #679, #9720, #2941 ) ;
#4141=DIRECTION ( 'NONE',  ( 0.000000000000000000, 0.000000000000000000, -1.000000000000000000 ) ) ;
#4145=EDGE_CURVE ( 'NONE', #8999, #6202, #4732, .T. ) ;
#4147=ORIENTED_EDGE ( 'NONE', *, *, #9159, .T. ) ;
#4148=DIRECTION ( 'NONE',  ( -0.000000000000000000, -1.000000000000000000, -0.000000000000000000 ) ) ;
#4149=EDGE_LOOP ( 'NONE', ( #8277, #5838, #2902, #6814 ) ) ;
#4151=AXIS2_PLACEMENT_3D ( 'NONE', #9377, #5630, #938 ) ;
#4153=CARTESIAN_POINT ( 'NONE',  ( -36.08344047792740383, 62.00000000000266454, -8.910509964045653319 ) ) ;
#4155=ORIENTED_EDGE ( 'NONE', *, *, #5924, .F. ) ;
#4156=LINE ( 'NONE', #1366, #4897 ) ;
#4165=ORIENTED_EDGE ( 'NONE', *, *, #837, .T. ) ;
#4169=DIRECTION ( 'NONE',  ( 0.000000000000000000, 0.000000000000000000, 1.000000000000000000 ) ) ;
#4173=DIRECTION ( 'NONE',  ( -0.000000000000000000, -1.000000000000000000, -0.000000000000000000 ) ) ;
#4179=CIRCLE ( 'NONE', #2574, 4.500000000000004441 ) ;
#4180=EDGE_LOOP ( 'NONE', ( #6065, #7503, #2069, #3214 ) ) ;
#4187=AXIS2_PLACEMENT_3D ( 'NONE', #1466, #6644, #1623 ) ;
#4193=EDGE_LOOP ( 'NONE', ( #6123, #804, #4601, #2502 ) ) ;
#4194=DIRECTION ( 'NONE',  ( 0.000000000000000000, 1.000000000000000000, 0.000000000000000000 ) ) ;
#4195=CARTESIAN_POINT ( 'NONE',  ( 5.562309845534932684, 61.99999999999999289, -28.56426808735048439 ) ) ;
#4196=EDGE_LOOP ( 'NONE', ( #4654, #766 ) ) ;
#4200=CIRCLE ( 'NONE', #9710, 2.500000000000002220 ) ;
#4205=DIRECTION ( 'NONE',  ( 0.000000000000000000, 0.000000000000000000, -1.000000000000000000 ) ) ;
#4207=VECTOR ( 'NONE', #1436, 1000.000000000000000 ) ;
#4209=ORIENTED_EDGE ( 'NONE', *, *, #9537, .T. ) ;
#4212=EDGE_LOOP ( 'NONE', ( #1986, #7139 ) ) ;
#4220=CARTESIAN_POINT ( 'NONE',  ( -33.06426808735054124, 60.99999999999999289, -5.562309845534581854 ) ) ;
#4229=DIRECTION ( 'NONE',  ( 0.000000000000000000, 0.000000000000000000, 1.000000000000000000 ) ) ;
#4233=ORIENTED_EDGE ( 'NONE', *, *, #3957, .F. ) ;
#4234=VERTEX_POINT ( 'NONE', #5065 ) ;
#4244=ORIENTED_EDGE ( 'NONE', *, *, #5215, .F. ) ;
#4251=EDGE_LOOP ( 'NONE', ( #7206, #675, #6435, #5574, #3442, #7969 ) ) ;
#4252=DIRECTION ( 'NONE',  ( -0.000000000000000000, 1.000000000000000000, -0.000000000000000000 ) ) ;
#4254=VERTEX_POINT ( 'NONE', #3581 ) ;
#4258=CARTESIAN_POINT ( 'NONE',  ( 16.29881421347312909, 60.99999999999999289, -2.568784777805685593 ) ) ;
#4261=EDGE_CURVE ( 'NONE', #7439, #64, #7246, .T. ) ;
#4277=DIRECTION ( 'NONE',  ( 0.000000000000000000, 0.000000000000000000, 1.000000000000000000 ) ) ;
#4281=DIRECTION ( 'NONE',  ( 0.000000000000000000, 0.000000000000000000, 1.000000000000000000 ) ) ;
#4287=DIRECTION ( 'NONE',  ( 0.000000000000000000, 1.000000000000000000, 0.000000000000000000 ) ) ;
#4292=CARTESIAN_POINT ( 'NONE',  ( 4.653657836759942730E-15, 0.000000000000000000, 38.00000000000000711 ) ) ;
#4294=CARTESIAN_POINT ( 'NONE',  ( 0.000000000000000000, 58.99999999999999289, -38.00000000000000711 ) ) ;
#4298=DIRECTION ( 'NONE',  ( 0.000000000000000000, 1.000000000000000000, 0.000000000000000000 ) ) ;
#4302=VECTOR ( 'NONE', #5530, 1000.000000000000000 ) ;
#4306=AXIS2_PLACEMENT_3D ( 'NONE', #980, #9432, #1131 ) ;
#4313=ORIENTED_EDGE ( 'NONE', *, *, #5344, .F. ) ;
#4325=ORIENTED_EDGE ( 'NONE', *, *, #991, .F. ) ;
#4330=CARTESIAN_POINT ( 'NONE',  ( 4.714890176717311093E-15, 61.99999999999999289, 37.00000000000001421 ) ) ;
#4331=EDGE_CURVE ( 'NONE', #1750, #1639, #6607, .T. ) ;
#4332=DIRECTION ( 'NONE',  ( 0.000000000000000000, 0.000000000000000000, 1.000000000000000000 ) ) ;
#4337=DIRECTION ( 'NONE',  ( 0.000000000000000000, -1.000000000000000000, 0.000000000000000000 ) ) ;
#4339=ORIENTED_EDGE ( 'NONE', *, *, #5211, .F. ) ;
#4350=FACE_BOUND ( 'NONE', #4591, .T. ) ;
#4358=ORIENTED_EDGE ( 'NONE', *, *, #749, .F. ) ;
#4366=VERTEX_POINT ( 'NONE', #6032 ) ;
#4371=FACE_OUTER_BOUND ( 'NONE', #3877, .T. ) ;
#4372=VERTEX_POINT ( 'NONE', #4527 ) ;
#4386=CARTESIAN_POINT ( 'NONE',  ( 0.000000000000000000, 52.29648987751954792, 0.000000000000000000 ) ) ;
#4387=EDGE_CURVE ( 'NONE', #1101, #9714, #4888, .T. ) ;
#4390=DIRECTION ( 'NONE',  ( 0.000000000000000000, 0.000000000000000000, 1.000000000000000000 ) ) ;
#4398=CARTESIAN_POINT ( 'NONE',  ( 0.000000000000000000, 60.99999999999999289, 0.000000000000000000 ) ) ;
#4399=EDGE_LOOP ( 'NONE', ( #949, #6609, #2826, #5162 ) ) ;
#4408=DIRECTION ( 'NONE',  ( -0.000000000000000000, 1.000000000000000000, -0.000000000000000000 ) ) ;
#4416=DIRECTION ( 'NONE',  ( -0.000000000000000000, -1.000000000000000000, -0.000000000000000000 ) ) ;
#4418=AXIS2_PLACEMENT_3D ( 'NONE', #8379, #4634, #6882 ) ;
#4419=AXIS2_PLACEMENT_3D ( 'NONE', #9713, #8135, #3735 ) ;
#4433=VECTOR ( 'NONE', #6044, 1000.000000000000000 ) ;
#4434=DIRECTION ( 'NONE',  ( -0.000000000000000000, -1.000000000000000000, -0.000000000000000000 ) ) ;
#4439=AXIS2_PLACEMENT_3D ( 'NONE', #8169, #5888, #5163 ) ;
#4442=FACE_OUTER_BOUND ( 'NONE', #4019, .T. ) ;
#4456=EDGE_CURVE ( 'NONE', #6645, #7858, #5201, .T. ) ;
#4460=LINE ( 'NONE', #5242, #2605 ) ;
#4464=CARTESIAN_POINT ( 'NONE',  ( -5.562309845534584518, 69.99999999999998579, 30.56426808735054124 ) ) ;
#4470=EDGE_LOOP ( 'NONE', ( #3171, #8151, #1476, #4625 ) ) ;
#4471=CARTESIAN_POINT ( 'NONE',  ( 0.000000000000000000, 61.99999999999999289, 0.000000000000000000 ) ) ;
#4476=CARTESIAN_POINT ( 'NONE',  ( 33.06426808735054124, 60.99999999999999289, 5.562309845534586294 ) ) ;
#4478=CYLINDRICAL_SURFACE ( 'NONE', #523, 40.00000000000000711 ) ;
#4482=DIRECTION ( 'NONE',  ( 0.000000000000000000, 0.000000000000000000, 1.000000000000000000 ) ) ;
#4491=CARTESIAN_POINT ( 'NONE',  ( -15.25056439471426195, 60.99999999999999289, 27.56211685706803038 ) ) ;
#4494=DIRECTION ( 'NONE',  ( 0.000000000000000000, 0.000000000000000000, -1.000000000000000000 ) ) ;
#4498=CIRCLE ( 'NONE', #4028, 37.00000000000000711 ) ;
#4506=ORIENTED_EDGE ( 'NONE', *, *, #4513, .T. ) ;
#4511=VERTEX_POINT ( 'NONE', #7751 ) ;
#4513=EDGE_CURVE ( 'NONE', #8621, #5790, #263, .T. ) ;
#4514=VERTEX_POINT ( 'NONE', #3301 ) ;
#4524=FACE_OUTER_BOUND ( 'NONE', #1983, .T. ) ;
#4526=EDGE_LOOP ( 'NONE', ( #1247, #8736 ) ) ;
#4527=CARTESIAN_POINT ( 'NONE',  ( -5.562309845534584518, 60.99999999999999289, 30.56426808735054124 ) ) ;
#4530=CARTESIAN_POINT ( 'NONE',  ( 0.000000000000000000, 61.99999999999999289, 0.000000000000000000 ) ) ;
#4534=CARTESIAN_POINT ( 'NONE',  ( 9.082100980773736509, 61.99999999999999289, -35.86802812777734317 ) ) ;
#4538=DIRECTION ( 'NONE',  ( -0.000000000000000000, -1.000000000000000000, -0.000000000000000000 ) ) ;
#4544=DIRECTION ( 'NONE',  ( -0.000000000000000000, -1.000000000000000000, -0.000000000000000000 ) ) ;
#4545=ORIENTED_EDGE ( 'NONE', *, *, #1305, .T. ) ;
#4550=FACE_OUTER_BOUND ( 'NONE', #6700, .T. ) ;
#4565=EDGE_CURVE ( 'NONE', #341, #7014, #4156, .T. ) ;
#4584=CARTESIAN_POINT ( 'NONE',  ( -8.634329568050702619, 61.97962948615073486, 36.36986309197412481 ) ) ;
#4591=EDGE_LOOP ( 'NONE', ( #3897, #7179 ) ) ;
#4595=AXIS2_PLACEMENT_3D ( 'NONE', #6727, #8031, #1267 ) ;
#4598=CARTESIAN_POINT ( 'NONE',  ( -5.137569555611031014, 60.99999999999999289, -32.59762842694632212 ) ) ;
#4601=ORIENTED_EDGE ( 'NONE', *, *, #6768, .T. ) ;
#4605=CARTESIAN_POINT ( 'NONE',  ( 3.903202352150908272, 61.96703986863185776, -37.25258870257768251 ) ) ;
#4612=CARTESIAN_POINT ( 'NONE',  ( 0.000000000000000000, 58.99999999999999289, 0.000000000000000000 ) ) ;
#4618=DIRECTION ( 'NONE',  ( -0.000000000000000000, 1.000000000000000000, -0.000000000000000000 ) ) ;
#4620=CIRCLE ( 'NONE', #976, 1.500000000000001332 ) ;
#4625=ORIENTED_EDGE ( 'NONE', *, *, #2723, .F. ) ;
#4626=CARTESIAN_POINT ( 'NONE',  ( 5.562309845534932684, 60.99999999999999289, -33.06426808735049150 ) ) ;
#4631=VECTOR ( 'NONE', #7026, 1000.000000000000000 ) ;
#4632=VERTEX_POINT ( 'NONE', #1138 ) ;
#4634=DIRECTION ( 'NONE',  ( -0.000000000000000000, -1.000000000000000000, -0.000000000000000000 ) ) ;
#4641=FACE_OUTER_BOUND ( 'NONE', #4180, .T. ) ;
#4644=EDGE_LOOP ( 'NONE', ( #1629, #8480, #2506, #7156 ) ) ;
#4649=CARTESIAN_POINT ( 'NONE',  ( 4.904043666719842598, 60.99999999999999289, 31.11591804390326743 ) ) ;
#4650=ORIENTED_EDGE ( 'NONE', *, *, #1775, .F. ) ;
#4651=CARTESIAN_POINT ( 'NONE',  ( 0.000000000000000000, 61.99999999999999289, -37.00000000000001421 ) ) ;
#4653=DIRECTION ( 'NONE',  ( 0.000000000000000000, 0.000000000000000000, 1.000000000000000000 ) ) ;
#4654=ORIENTED_EDGE ( 'NONE', *, *, #3911, .T. ) ;
#4656=EDGE_LOOP ( 'NONE', ( #4165, #1778, #4767, #3391 ) ) ;
#4658=VECTOR ( 'NONE', #2237, 1000.000000000000000 ) ;
#4659=DIRECTION ( 'NONE',  ( 0.000000000000000000, 0.000000000000000000, -1.000000000000000000 ) ) ;
#4662=ORIENTED_EDGE ( 'NONE', *, *, #5037, .F. ) ;
#4664=CARTESIAN_POINT ( 'NONE',  ( -3.903202352150655585, 61.96703986863184355, 37.25258870257768962 ) ) ;
#4669=CIRCLE ( 'NONE', #3238, 4.500000000000004441 ) ;
#4675=AXIS2_PLACEMENT_3D ( 'NONE', #1846, #4863, #2629 ) ;
#4678=FACE_OUTER_BOUND ( 'NONE', #7061, .T. ) ;
#4683=ORIENTED_EDGE ( 'NONE', *, *, #1832, .T. ) ;
#4691=LINE ( 'NONE', #974, #1968 ) ;
#4692=EDGE_CURVE ( 'NONE', #64, #7439, #172, .T. ) ;
#4694=EDGE_CURVE ( 'NONE', #9299, #4234, #8521, .T. ) ;
#4699=FACE_BOUND ( 'NONE', #543, .T. ) ;
#4702=DIRECTION ( 'NONE',  ( 0.000000000000000000, 0.000000000000000000, 1.000000000000000000 ) ) ;
#4703=CARTESIAN_POINT ( 'NONE',  ( -27.56211685706797709, 61.99999999999999289, -15.25056439471436676 ) ) ;
#4706=DIRECTION ( 'NONE',  ( 0.000000000000000000, 0.000000000000000000, 1.000000000000000000 ) ) ;
#4707=CARTESIAN_POINT ( 'NONE',  ( -15.97678174684350871, 60.99999999999999289, 28.87459861216650836 ) ) ;
#4709=ORIENTED_EDGE ( 'NONE', *, *, #5282, .T. ) ;
#4711=CARTESIAN_POINT ( 'NONE',  ( -3.332326962091669120, 61.99999999999999289, 36.97859170863238631 ) ) ;
#4722=CYLINDRICAL_SURFACE ( 'NONE', #637, 1.500000000000001332 ) ;
#4723=DIRECTION ( 'NONE',  ( -0.000000000000000000, 1.000000000000000000, 0.000000000000000000 ) ) ;
#4724=ORIENTED_EDGE ( 'NONE', *, *, #8103, .F. ) ;
#4727=DIRECTION ( 'NONE',  ( 0.000000000000000000, 0.000000000000000000, 1.000000000000000000 ) ) ;
#4730=ORIENTED_EDGE ( 'NONE', *, *, #3124, .F. ) ;
#4732=CIRCLE ( 'NONE', #9618, 1.500000000000001332 ) ;
#4741=CARTESIAN_POINT ( 'NONE',  ( 37.54740336257584232, 61.81808349686849624, 6.037872445562960877 ) ) ;
#4745=CARTESIAN_POINT ( 'NONE',  ( 0.000000000000000000, 60.99999999999999289, 0.000000000000000000 ) ) ;
#4747=CARTESIAN_POINT ( 'NONE',  ( -37.55900191124520404, 61.85658167520826822, -5.210294541070858543 ) ) ;
#4748=VERTEX_POINT ( 'NONE', #89 ) ;
#4750=DIRECTION ( 'NONE',  ( -0.000000000000000000, -1.000000000000000000, -0.000000000000000000 ) ) ;
#4758=ADVANCED_FACE ( 'NONE', ( #5368 ), #6140, .F. ) ;
#4765=VERTEX_POINT ( 'NONE', #4534 ) ;
#4767=ORIENTED_EDGE ( 'NONE', *, *, #8796, .F. ) ;
#4781=DIRECTION ( 'NONE',  ( 0.000000000000000000, 1.000000000000000000, 0.000000000000000000 ) ) ;
#4786=CIRCLE ( 'NONE', #2853, 2.500000000000002220 ) ;
#4793=CYLINDRICAL_SURFACE ( 'NONE', #3699, 1.500000000000001332 ) ;
#4795=CARTESIAN_POINT ( 'NONE',  ( -5.562309845534700870, 60.99999999999999289, 28.56426808735051992 ) ) ;
#4800=DIRECTION ( 'NONE',  ( 0.000000000000000000, 1.000000000000000000, 0.000000000000000000 ) ) ;
#4802=CARTESIAN_POINT ( 'NONE',  ( -5.562309845534700870, 61.99999999999999289, 28.56426808735051992 ) ) ;
#4804=ORIENTED_EDGE ( 'NONE', *, *, #5225, .F. ) ;
#4808=ADVANCED_FACE ( 'NONE', ( #3888 ), #4722, .F. ) ;
#4812=ORIENTED_EDGE ( 'NONE', *, *, #7761, .F. ) ;
#4814=ADVANCED_FACE ( 'NONE', ( #6830 ), #5420, .T. ) ;
#4819=VECTOR ( 'NONE', #753, 1000.000000000000000 ) ;
#4820=DIRECTION ( 'NONE',  ( -0.000000000000000000, 1.000000000000000000, -0.000000000000000000 ) ) ;
#4828=ORIENTED_EDGE ( 'NONE', *, *, #350, .T. ) ;
#4845=AXIS2_PLACEMENT_3D ( 'NONE', #7911, #8506, #1691 ) ;
#4848=CARTESIAN_POINT ( 'NONE',  ( 0.000000000000000000, 0.000000000000000000, 0.000000000000000000 ) ) ;
#4851=LINE ( 'NONE', #3159, #3576 ) ;
#4856=DIRECTION ( 'NONE',  ( -0.000000000000000000, -1.000000000000000000, -0.000000000000000000 ) ) ;
#4862=EDGE_CURVE ( 'NONE', #6026, #1665, #6619, .T. ) ;
#4863=DIRECTION ( 'NONE',  ( 0.000000000000000000, 1.000000000000000000, 0.000000000000000000 ) ) ;
#4870=FACE_OUTER_BOUND ( 'NONE', #5779, .T. ) ;
#4875=CARTESIAN_POINT ( 'NONE',  ( 5.137569555611264605, 61.99999999999999289, 34.09762842694627949 ) ) ;
#4880=ORIENTED_EDGE ( 'NONE', *, *, #9311, .T. ) ;
#4881=CARTESIAN_POINT ( 'NONE',  ( 5.902069945235307813, 61.82045560759793545, -37.56426808735049860 ) ) ;
#4888=CIRCLE ( 'NONE', #632, 1.500000000000001332 ) ;
#4897=VECTOR ( 'NONE', #4337, 1000.000000000000000 ) ;
#4900=CARTESIAN_POINT ( 'NONE',  ( -15.97678174684350871, 60.99999999999999289, 30.37459861216651191 ) ) ;
#4903=DIRECTION ( 'NONE',  ( 0.000000000000000000, 1.000000000000000000, 0.000000000000000000 ) ) ;
#4912=DIRECTION ( 'NONE',  ( -0.000000000000000000, 1.000000000000000000, -0.000000000000000000 ) ) ;
#4921=DIRECTION ( 'NONE',  ( 0.000000000000000000, 0.000000000000000000, -1.000000000000000000 ) ) ;
#4924=CIRCLE ( 'NONE', #7918, 2.500000000000002220 ) ;
#4925=DIRECTION ( 'NONE',  ( 0.000000000000000000, 0.000000000000000000, 1.000000000000000000 ) ) ;
#4929=EDGE_CURVE ( 'NONE', #3340, #5097, #6150, .T. ) ;
#4932=CARTESIAN_POINT ( 'NONE',  ( 5.562309845534932684, 60.99999999999999289, -28.56426808735048439 ) ) ;
#4941=DIRECTION ( 'NONE',  ( 0.000000000000000000, 0.000000000000000000, 1.000000000000000000 ) ) ;
#4942=VECTOR ( 'NONE', #6941, 1000.000000000000000 ) ;
#4975=CIRCLE ( 'NONE', #7334, 37.00000000000000711 ) ;
#4991=FACE_BOUND ( 'NONE', #1613, .T. ) ;
#4996=ORIENTED_EDGE ( 'NONE', *, *, #4929, .T. ) ;
#5001=ADVANCED_FACE ( 'NONE', ( #2484 ), #246, .F. ) ;
#5011=FACE_OUTER_BOUND ( 'NONE', #4656, .T. ) ;
#5020=DIRECTION ( 'NONE',  ( 0.000000000000000000, 1.000000000000000000, 0.000000000000000000 ) ) ;
#5035=FACE_BOUND ( 'NONE', #7965, .T. ) ;
#5037=EDGE_CURVE ( 'NONE', #4366, #4234, #6250, .T. ) ;
#5048=ADVANCED_FACE ( 'NONE', ( #9080 ), #2297, .T. ) ;
#5060=AXIS2_PLACEMENT_3D ( 'NONE', #9655, #5020, #670 ) ;
#5065=CARTESIAN_POINT ( 'NONE',  ( -5.562309845534584518, 59.99999999999999289, 35.56426808735054834 ) ) ;
#5077=CARTESIAN_POINT ( 'NONE',  ( 5.137569555611264605, 60.99999999999999289, 32.59762842694627949 ) ) ;
#5082=FACE_BOUND ( 'NONE', #6965, .T. ) ;
#5084=EDGE_LOOP ( 'NONE', ( #7313, #6338, #1053, #3798 ) ) ;
#5088=CIRCLE ( 'NONE', #9353, 27.99999999999999289 ) ;
#5089=ORIENTED_EDGE ( 'NONE', *, *, #2519, .T. ) ;
#5097=VERTEX_POINT ( 'NONE', #3088 ) ;
#5102=DIRECTION ( 'NONE',  ( 0.000000000000000000, 0.000000000000000000, 1.000000000000000000 ) ) ;
#5103=B_SPLINE_CURVE_WITH_KNOTS ( 'NONE', 3,
 ( #5452, #1695, #3116, #8411, #4664, #7575, #4711, #3014 ),
 .UNSPECIFIED., .F., .F.,
 ( 4, 2, 2, 4 ),
 ( 0.007099638519839682714, 0.008372149287075627763, 0.009008404670693602456, 0.009644660054311575414 ),
 .UNSPECIFIED. ) ;
#5111=VERTEX_POINT ( 'NONE', #7080 ) ;
#5117=CARTESIAN_POINT ( 'NONE',  ( 27.56211685706808723, 60.99999999999999289, 15.25056439471416780 ) ) ;
#5118=AXIS2_PLACEMENT_3D ( 'NONE', #6444, #9474, #2692 ) ;
#5120=EDGE_CURVE ( 'NONE', #8580, #3849, #2675, .T. ) ;
#5140=PLANE ( 'NONE',  #9383 ) ;
#5153=VERTEX_POINT ( 'NONE', #2683 ) ;
#5156=CARTESIAN_POINT ( 'NONE',  ( 15.25056439471407188, 60.99999999999999289, -27.56211685706813341 ) ) ;
#5162=ORIENTED_EDGE ( 'NONE', *, *, #5762, .F. ) ;
#5163=DIRECTION ( 'NONE',  ( 0.000000000000000000, 0.000000000000000000, -1.000000000000000000 ) ) ;
#5164=VERTEX_POINT ( 'NONE', #6487 ) ;
#5168=DIRECTION ( 'NONE',  ( 1.000000000000000000, 0.000000000000000000, 0.000000000000000000 ) ) ;
#5169=CARTESIAN_POINT ( 'NONE',  ( 0.000000000000000000, 61.99999999999999289, 0.000000000000000000 ) ) ;
#5176=FACE_OUTER_BOUND ( 'NONE', #359, .T. ) ;
#5181=CARTESIAN_POINT ( 'NONE',  ( 0.000000000000000000, 0.000000000000000000, -38.00000000000000711 ) ) ;
#5186=ORIENTED_EDGE ( 'NONE', *, *, #1811, .T. ) ;
#5188=LINE ( 'NONE', #2199, #1506 ) ;
#5190=ORIENTED_EDGE ( 'NONE', *, *, #526, .T. ) ;
#5196=ORIENTED_EDGE ( 'NONE', *, *, #991, .T. ) ;
#5201=CIRCLE ( 'NONE', #6448, 2.500000000000002220 ) ;
#5209=DIRECTION ( 'NONE',  ( 0.000000000000000000, 1.000000000000000000, 0.000000000000000000 ) ) ;
#5210=FACE_OUTER_BOUND ( 'NONE', #4196, .T. ) ;
#5211=EDGE_CURVE ( 'NONE', #7361, #849, #1740, .T. ) ;
#5212=CYLINDRICAL_SURFACE ( 'NONE', #8446, 1.499999999999999556 ) ;
#5214=VECTOR ( 'NONE', #1903, 1000.000000000000000 ) ;
#5215=EDGE_CURVE ( 'NONE', #8835, #5097, #2532, .T. ) ;
#5225=EDGE_CURVE ( 'NONE', #4748, #5814, #4089, .T. ) ;
#5234=AXIS2_PLACEMENT_3D ( 'NONE', #5077, #8087, #7350 ) ;
#5241=ORIENTED_EDGE ( 'NONE', *, *, #5120, .F. ) ;
#5242=CARTESIAN_POINT ( 'NONE',  ( -33.06426808735054124, 60.99999999999999289, -1.062309845534581632 ) ) ;
#5250=VECTOR ( 'NONE', #3884, 1000.000000000000000 ) ;
#5253=ORIENTED_EDGE ( 'NONE', *, *, #8476, .F. ) ;
#5257=UNCERTAINTY_MEASURE_WITH_UNIT (LENGTH_MEASURE( 1.000000000000000082E-05 ), #7163, 'distance_accuracy_value', 'NONE');
#5275=TOROIDAL_SURFACE ( 'NONE', #245, 37.00000000000000711, 1.000000000000000888 ) ;
#5281=ADVANCED_FACE ( 'NONE', ( #9607, #5210 ), #2175, .T. ) ;
#5282=EDGE_CURVE ( 'NONE', #2645, #7767, #8049, .T. ) ;
#5285=DIRECTION ( 'NONE',  ( 0.000000000000000000, 0.000000000000000000, -1.000000000000000000 ) ) ;
#5286=DIRECTION ( 'NONE',  ( -0.000000000000000000, -1.000000000000000000, -0.000000000000000000 ) ) ;
#5288=AXIS2_PLACEMENT_3D ( 'NONE', #2715, #2812, #1248 ) ;
#5292=AXIS2_PLACEMENT_3D ( 'NONE', #4027, #4820, #8624 ) ;
#5300=ORIENTED_EDGE ( 'NONE', *, *, #2477, .F. ) ;
#5301=EDGE_CURVE ( 'NONE', #7014, #5814, #9317, .T. ) ;
#5310=ORIENTED_EDGE ( 'NONE', *, *, #4331, .F. ) ;
#5311=DIRECTION ( 'NONE',  ( -0.000000000000000000, 1.000000000000000000, 0.000000000000000000 ) ) ;
#5318=CARTESIAN_POINT ( 'NONE',  ( 0.000000000000000000, 61.99999999999999289, 0.000000000000000000 ) ) ;
#5319=EDGE_CURVE ( 'NONE', #1356, #4632, #8840, .T. ) ;
#5322=VERTEX_POINT ( 'NONE', #4330 ) ;
#5328=ORIENTED_EDGE ( 'NONE', *, *, #6175, .T. ) ;
#5334=DIRECTION ( 'NONE',  ( 0.000000000000000000, 0.000000000000000000, 1.000000000000000000 ) ) ;
#5344=EDGE_CURVE ( 'NONE', #903, #5641, #6538, .T. ) ;
#5355=ADVANCED_FACE ( 'NONE', ( #1403 ), #2831, .T. ) ;
#5356=ORIENTED_EDGE ( 'NONE', *, *, #8610, .T. ) ;
#5360=ORIENTED_EDGE ( 'NONE', *, *, #5826, .T. ) ;
#5363=CARTESIAN_POINT ( 'NONE',  ( -28.87459861216645862, 61.99999999999999289, -14.47678174684361352 ) ) ;
#5368=FACE_OUTER_BOUND ( 'NONE', #9649, .T. ) ;
#5383=ORIENTED_EDGE ( 'NONE', *, *, #4387, .F. ) ;
#5387=AXIS2_PLACEMENT_3D ( 'NONE', #6394, #2040, #5754 ) ;
#5395=DIRECTION ( 'NONE',  ( 0.000000000000000000, 1.000000000000000000, 0.000000000000000000 ) ) ;
#5398=CYLINDRICAL_SURFACE ( 'NONE', #7510, 31.49999999999999289 ) ;
#5403=DIRECTION ( 'NONE',  ( -0.000000000000000000, 1.000000000000000000, -0.000000000000000000 ) ) ;
#5411=CIRCLE ( 'NONE', #211, 40.00000000000000711 ) ;
#5420=PLANE ( 'NONE',  #8988 ) ;
#5451=DIRECTION ( 'NONE',  ( -0.000000000000000000, 1.000000000000000000, -0.000000000000000000 ) ) ;
#5452=CARTESIAN_POINT ( 'NONE',  ( -5.562309845534701758, 61.83753588906734677, 37.56426808735052703 ) ) ;
#5454=AXIS2_PLACEMENT_3D ( 'NONE', #1949, #6290, #4925 ) ;
#5458=ORIENTED_EDGE ( 'NONE', *, *, #3540, .T. ) ;
#5465=ADVANCED_FACE ( 'NONE', ( #3172 ), #2332, .F. ) ;
#5492=DIRECTION ( 'NONE',  ( 0.000000000000000000, 1.000000000000000000, 0.000000000000000000 ) ) ;
#5495=CYLINDRICAL_SURFACE ( 'NONE', #7191, 38.00000000000000711 ) ;
#5511=CYLINDRICAL_SURFACE ( 'NONE', #6023, 2.500000000000002220 ) ;
#5520=CIRCLE ( 'NONE', #4418, 31.49999999999999289 ) ;
#5525=EDGE_LOOP ( 'NONE', ( #6295, #3973 ) ) ;
#5526=DIRECTION ( 'NONE',  ( 0.000000000000000000, 0.000000000000000000, 1.000000000000000000 ) ) ;
#5527=CARTESIAN_POINT ( 'NONE',  ( 35.86802812777743554, 61.99999999999999289, 9.082100980773358145 ) ) ;
#5530=DIRECTION ( 'NONE',  ( -0.000000000000000000, 1.000000000000000000, -0.000000000000000000 ) ) ;
#5532=AXIS2_PLACEMENT_3D ( 'NONE', #444, #9425, #7935 ) ;
#5534=CARTESIAN_POINT ( 'NONE',  ( -37.42097066196858179, 61.92370482830305889, -4.403127714044224206 ) ) ;
#5542=ORIENTED_EDGE ( 'NONE', *, *, #8666, .F. ) ;
#5548=DIRECTION ( 'NONE',  ( 0.000000000000000000, 0.000000000000000000, 1.000000000000000000 ) ) ;
#5560=AXIS2_PLACEMENT_3D ( 'NONE', #6852, #2999, #7 ) ;
#5564=CARTESIAN_POINT ( 'NONE',  ( 15.25056439471407188, 60.99999999999999289, -27.56211685706813341 ) ) ;
#5565=LINE ( 'NONE', #1170, #2115 ) ;
#5569=ORIENTED_EDGE ( 'NONE', *, *, #8502, .T. ) ;
#5572=DIRECTION ( 'NONE',  ( 0.000000000000000000, 1.000000000000000000, 0.000000000000000000 ) ) ;
#5574=ORIENTED_EDGE ( 'NONE', *, *, #1061, .T. ) ;
#5575=CARTESIAN_POINT ( 'NONE',  ( -15.97678174684350871, 60.99999999999999289, 28.87459861216650836 ) ) ;
#5579=DIRECTION ( 'NONE',  ( 0.000000000000000000, 0.000000000000000000, 1.000000000000000000 ) ) ;
#5580=ADVANCED_FACE ( 'NONE', ( #3764 ), #4793, .F. ) ;
#5591=CIRCLE ( 'NONE', #2584, 4.500000000000005329 ) ;
#5595=ORIENTED_EDGE ( 'NONE', *, *, #6490, .T. ) ;
#5628=EDGE_LOOP ( 'NONE', ( #6583, #4006, #3768, #3176 ) ) ;
#5630=DIRECTION ( 'NONE',  ( 0.000000000000000000, 1.000000000000000000, 0.000000000000000000 ) ) ;
#5641=VERTEX_POINT ( 'NONE', #9478 ) ;
#5643=DIRECTION ( 'NONE',  ( 1.000000000000000000, 0.000000000000000000, 1.079383496163345602E-14 ) ) ;
#5644=EDGE_CURVE ( 'NONE', #1356, #5699, #3055, .T. ) ;
#5646=CARTESIAN_POINT ( 'NONE',  ( -28.87459861216645862, 60.99999999999999289, -14.47678174684361352 ) ) ;
#5650=EDGE_LOOP ( 'NONE', ( #8305, #1388, #796, #6943 ) ) ;
#5657=EDGE_CURVE ( 'NONE', #8683, #7884, #7098, .T. ) ;
#5660=EDGE_LOOP ( 'NONE', ( #9283, #2577 ) ) ;
#5673=EDGE_LOOP ( 'NONE', ( #7278, #8290, #7882, #9641, #4545, #8058, #6154, #6909, #3660 ) ) ;
#5683=EDGE_LOOP ( 'NONE', ( #4233, #6471, #9463, #7909, #4812 ) ) ;
#5692=DIRECTION ( 'NONE',  ( 0.000000000000000000, 0.000000000000000000, -1.000000000000000000 ) ) ;
#5694=VERTEX_POINT ( 'NONE', #5720 ) ;
#5699=VERTEX_POINT ( 'NONE', #3492 ) ;
#5704=EDGE_CURVE ( 'NONE', #5699, #64, #1134, .T. ) ;
#5720=CARTESIAN_POINT ( 'NONE',  ( -5.371095444502437921, 60.99999999999999289, -34.07933880998933773 ) ) ;
#5726=EDGE_LOOP ( 'NONE', ( #6134, #6213, #6712, #8549, #3609, #7468, #6615, #747, #1401, #9604, #935, #5310, #1130, #703, #88, #3094 ) ) ;
#5727=FACE_BOUND ( 'NONE', #8955, .T. ) ;
#5729=AXIS2_PLACEMENT_3D ( 'NONE', #2591, #4194, #8492 ) ;
#5745=AXIS2_PLACEMENT_3D ( 'NONE', #8738, #3400, #8786 ) ;
#5754=DIRECTION ( 'NONE',  ( 0.000000000000000000, 0.000000000000000000, -1.000000000000000000 ) ) ;
#5762=EDGE_CURVE ( 'NONE', #7580, #7439, #8231, .T. ) ;
#5770=( NAMED_UNIT ( * ) PLANE_ANGLE_UNIT ( ) SI_UNIT ( $, .RADIAN. ) );
#5771=TOROIDAL_SURFACE ( 'NONE', #1507, 37.00000000000000711, 3.000000000000002665 ) ;
#5779=EDGE_LOOP ( 'NONE', ( #6275, #153 ) ) ;
#5787=PLANE ( 'NONE',  #8131 ) ;
#5790=VERTEX_POINT ( 'NONE', #7447 ) ;
#5792=CARTESIAN_POINT ( 'NONE',  ( 33.06426808735054124, 60.99999999999999289, 1.062309845534581632 ) ) ;
#5802=ORIENTED_EDGE ( 'NONE', *, *, #3586, .F. ) ;
#5814=VERTEX_POINT ( 'NONE', #3639 ) ;
#5815=FACE_OUTER_BOUND ( 'NONE', #4024, .T. ) ;
#5826=EDGE_CURVE ( 'NONE', #8835, #7681, #2261, .T. ) ;
#5827=CARTESIAN_POINT ( 'NONE',  ( 5.562309845534588959, 59.99999999999999289, -35.56426808735054834 ) ) ;
#5830=DIRECTION ( 'NONE',  ( -0.000000000000000000, 1.000000000000000000, -0.000000000000000000 ) ) ;
#5836=VERTEX_POINT ( 'NONE', #9230 ) ;
#5837=DIRECTION ( 'NONE',  ( -0.000000000000000000, 1.000000000000000000, -0.000000000000000000 ) ) ;
#5838=ORIENTED_EDGE ( 'NONE', *, *, #9280, .F. ) ;
#5844=CYLINDRICAL_SURFACE ( 'NONE', #4439, 27.99999999999999289 ) ;
#5853=PRODUCT_DEFINITION_FORMATION_WITH_SPECIFIED_SOURCE ( 'ANY', '', #786, .NOT_KNOWN. ) ;
#5861=AXIS2_PLACEMENT_3D ( 'NONE', #8653, #4116, #9296 ) ;
#5864=DIRECTION ( 'NONE',  ( 0.000000000000000000, 1.000000000000000000, 0.000000000000000000 ) ) ;
#5875=EDGE_LOOP ( 'NONE', ( #5802, #6590, #2228, #9726 ) ) ;
#5877=ADVANCED_FACE ( 'NONE', ( #8338 ), #1713, .F. ) ;
#5881=CARTESIAN_POINT ( 'NONE',  ( -33.06426808735054124, 60.99999999999999289, -5.562309845534586294 ) ) ;
#5888=DIRECTION ( 'NONE',  ( -0.000000000000000000, -1.000000000000000000, -0.000000000000000000 ) ) ;
#5899=CIRCLE ( 'NONE', #8437, 40.00000000000000711 ) ;
#5900=CARTESIAN_POINT ( 'NONE',  ( -8.871504613779674031, 62.00000000000265743, 36.13240710991937021 ) ) ;
#5907=AXIS2_PLACEMENT_3D ( 'NONE', #4612, #5968, #4659 ) ;
#5909=CIRCLE ( 'NONE', #2446, 1.500000000000003109 ) ;
#5911=AXIS2_PLACEMENT_3D ( 'NONE', #8661, #4173, #5692 ) ;
#5913=EDGE_LOOP ( 'NONE', ( #6603, #2468 ) ) ;
#5919=AXIS2_PLACEMENT_3D ( 'NONE', #1140, #4800, #2410 ) ;
#5921=ORIENTED_EDGE ( 'NONE', *, *, #224, .T. ) ;
#5924=EDGE_CURVE ( 'NONE', #6645, #5153, #8529, .T. ) ;
#5925=ORIENTED_EDGE ( 'NONE', *, *, #9158, .F. ) ;
#5934=B_SPLINE_CURVE_WITH_KNOTS ( 'NONE', 3,
 ( #8499, #4153, #4056, #9437, #7101, #4103, #9288, #2649, #349, #6260, #1137, #4747, #400, #5534, #3353, #3405, #9380, #7046 ),
 .UNSPECIFIED., .F., .F.,
 ( 4, 2, 2, 2, 2, 2, 2, 2, 4 ),
 ( 0.003057178249550605680, 0.003880613475145725487, 0.004704048700740845294, 0.005527483926335964234, 0.006350919151931084042, 0.007174354377526204717, 0.007997789603121323657, 0.008821224828716443464, 0.009644660054311565006 ),
 .UNSPECIFIED. ) ;
#5939=CARTESIAN_POINT ( 'NONE',  ( 5.371095444502685723, 61.99999999999999289, 34.07933880998929510 ) ) ;
#5940=CARTESIAN_POINT ( 'NONE',  ( 33.06426808735054124, 61.99999999999999289, 5.562309845534586294 ) ) ;
#5952=DIRECTION ( 'NONE',  ( 0.000000000000000000, 0.000000000000000000, 1.000000000000000000 ) ) ;
#5962=CARTESIAN_POINT ( 'NONE',  ( 33.06426808735054124, 60.99999999999999289, 1.062309845534581632 ) ) ;
#5966=ORIENTED_EDGE ( 'NONE', *, *, #6545, .F. ) ;
#5968=DIRECTION ( 'NONE',  ( -0.000000000000000000, -1.000000000000000000, -0.000000000000000000 ) ) ;
#5972=DIRECTION ( 'NONE',  ( 0.000000000000000000, 0.000000000000000000, 1.000000000000000000 ) ) ;
#5973=AXIS2_PLACEMENT_3D ( 'NONE', #1499, #2173, #1450 ) ;
#5980=EDGE_CURVE ( 'NONE', #6704, #8580, #4691, .T. ) ;
#5992=ORIENTED_EDGE ( 'NONE', *, *, #35, .T. ) ;
#6000=LINE ( 'NONE', #4491, #1327 ) ;
#6001=EDGE_CURVE ( 'NONE', #4765, #7319, #4975, .T. ) ;
#6002=VERTEX_POINT ( 'NONE', #4091 ) ;
#6005=ORIENTED_EDGE ( 'NONE', *, *, #8452, .F. ) ;
#6008=CARTESIAN_POINT ( 'NONE',  ( 0.000000000000000000, 58.99999999999999289, 0.000000000000000000 ) ) ;
#6012=SHAPE_DEFINITION_REPRESENTATION ( #8687, #2928 ) ;
#6013=CIRCLE ( 'NONE', #4151, 1.500000000000001332 ) ;
#6015=CARTESIAN_POINT ( 'NONE',  ( 33.06426808735054124, 69.99999999999998579, 3.062309845534584074 ) ) ;
#6021=DIRECTION ( 'NONE',  ( -0.000000000000000000, 1.000000000000000000, -0.000000000000000000 ) ) ;
#6022=LINE ( 'NONE', #3816, #6493 ) ;
#6023=AXIS2_PLACEMENT_3D ( 'NONE', #9218, #6879, #8327 ) ;
#6026=VERTEX_POINT ( 'NONE', #1123 ) ;
#6029=CIRCLE ( 'NONE', #7300, 4.500000000000004441 ) ;
#6032=CARTESIAN_POINT ( 'NONE',  ( -5.562309845534584518, 60.99999999999999289, 35.56426808735054834 ) ) ;
#6035=ORIENTED_EDGE ( 'NONE', *, *, #2251, .T. ) ;
#6038=ADVANCED_FACE ( 'NONE', ( #8775 ), #7236, .F. ) ;
#6044=DIRECTION ( 'NONE',  ( 0.000000000000000000, -1.000000000000000000, 0.000000000000000000 ) ) ;
#6057=VERTEX_POINT ( 'NONE', #4875 ) ;
#6065=ORIENTED_EDGE ( 'NONE', *, *, #7259, .T. ) ;
#6074=DIRECTION ( 'NONE',  ( 0.000000000000000000, 1.000000000000000000, 0.000000000000000000 ) ) ;
#6075=CARTESIAN_POINT ( 'NONE',  ( -5.562309845534700870, 60.99999999999999289, 28.56426808735051992 ) ) ;
#6081=AXIS2_PLACEMENT_3D ( 'NONE', #9738, #5395, #124 ) ;
#6109=CARTESIAN_POINT ( 'NONE',  ( -33.06426808735054124, 60.99999999999999289, -1.062309845534581632 ) ) ;
#6118=CARTESIAN_POINT ( 'NONE',  ( 32.59762842694625817, 60.99999999999999289, -5.137569555611371186 ) ) ;
#6119=EDGE_CURVE ( 'NONE', #6057, #1263, #2752, .T. ) ;
#6123=ORIENTED_EDGE ( 'NONE', *, *, #9244, .F. ) ;
#6124=CARTESIAN_POINT ( 'NONE',  ( 30.18708036726505028, 60.99999999999999289, 16.70299909897265778 ) ) ;
#6125=EDGE_CURVE ( 'NONE', #6002, #1252, #5565, .T. ) ;
#6128=DIRECTION ( 'NONE',  ( 0.000000000000000000, -0.000000000000000000, 1.000000000000000000 ) ) ;
#6134=ORIENTED_EDGE ( 'NONE', *, *, #2384, .F. ) ;
#6140=CYLINDRICAL_SURFACE ( 'NONE', #8366, 4.500000000000004441 ) ;
#6150=CIRCLE ( 'NONE', #3309, 1.500000000000001332 ) ;
#6154=ORIENTED_EDGE ( 'NONE', *, *, #3650, .F. ) ;
#6158=CARTESIAN_POINT ( 'NONE',  ( 37.01190402608325059, 62.00000000000000711, 3.384896555618068348 ) ) ;
#6162=EDGE_LOOP ( 'NONE', ( #6863, #9405, #5196, #2465, #3016 ) ) ;
#6164=CARTESIAN_POINT ( 'NONE',  ( -33.06426808735054124, 61.99999999999999289, -10.06230984553459251 ) ) ;
#6174=CIRCLE ( 'NONE', #7448, 2.499999999999998668 ) ;
#6175=EDGE_CURVE ( 'NONE', #5322, #7811, #4498, .T. ) ;
#6183=CIRCLE ( 'NONE', #3190, 1.499999999999999556 ) ;
#6187=ADVANCED_FACE ( 'NONE', ( #8080 ), #5212, .F. ) ;
#6190=CARTESIAN_POINT ( 'NONE',  ( -15.97678174684350871, 60.99999999999999289, 28.87459861216650836 ) ) ;
#6201=CARTESIAN_POINT ( 'NONE',  ( 33.06426808735054124, 60.99999999999999289, 5.562309845534586294 ) ) ;
#6202=VERTEX_POINT ( 'NONE', #5117 ) ;
#6206=ORIENTED_EDGE ( 'NONE', *, *, #7147, .F. ) ;
#6213=ORIENTED_EDGE ( 'NONE', *, *, #6175, .F. ) ;
#6229=DIRECTION ( 'NONE',  ( 0.000000000000000000, 0.000000000000000000, -1.000000000000000000 ) ) ;
#6241=ORIENTED_EDGE ( 'NONE', *, *, #1725, .F. ) ;
#6244=DIRECTION ( 'NONE',  ( -0.000000000000000000, -1.000000000000000000, -0.000000000000000000 ) ) ;
#6247=AXIS2_PLACEMENT_3D ( 'NONE', #7360, #8744, #3413 ) ;
#6250=LINE ( 'NONE', #9275, #4433 ) ;
#6252=CARTESIAN_POINT ( 'NONE',  ( -33.06426808735054124, 69.99999999999998579, -3.062309845534580077 ) ) ;
#6256=CARTESIAN_POINT ( 'NONE',  ( 6.235648121649441045, 61.81426382726520075, -37.52627707316309369 ) ) ;
#6260=CARTESIAN_POINT ( 'NONE',  ( -37.54740336257584232, 61.81808349686849624, -6.037872445562960877 ) ) ;
#6264=FACE_OUTER_BOUND ( 'NONE', #1435, .T. ) ;
#6267=ORIENTED_EDGE ( 'NONE', *, *, #2231, .F. ) ;
#6271=CARTESIAN_POINT ( 'NONE',  ( -36.86535760663189620, 61.99999999999999289, -3.153634179030289530 ) ) ;
#6275=ORIENTED_EDGE ( 'NONE', *, *, #3332, .T. ) ;
#6282=ORIENTED_EDGE ( 'NONE', *, *, #9268, .F. ) ;
#6284=ORIENTED_EDGE ( 'NONE', *, *, #5301, .F. ) ;
#6287=DIRECTION ( 'NONE',  ( 0.000000000000000000, 0.000000000000000000, 1.000000000000000000 ) ) ;
#6290=DIRECTION ( 'NONE',  ( 0.000000000000000000, 1.000000000000000000, 0.000000000000000000 ) ) ;
#6295=ORIENTED_EDGE ( 'NONE', *, *, #7649, .T. ) ;
#6297=APPLICATION_CONTEXT ( 'automotive_design' ) ;
#6299=ORIENTED_EDGE ( 'NONE', *, *, #2424, .F. ) ;
#6300=LINE ( 'NONE', #3193, #388 ) ;
#6306=CARTESIAN_POINT ( 'NONE',  ( 0.000000000000000000, 58.99999999999999289, 0.000000000000000000 ) ) ;
#6308=CARTESIAN_POINT ( 'NONE',  ( 4.898587196589413815E-15, 58.99999999999999289, 40.00000000000000711 ) ) ;
#6314=AXIS2_PLACEMENT_3D ( 'NONE', #9654, #2830, #5168 ) ;
#6316=DIRECTION ( 'NONE',  ( -0.000000000000000000, 1.000000000000000000, -0.000000000000000000 ) ) ;
#6320=DIRECTION ( 'NONE',  ( 0.000000000000000000, 0.000000000000000000, -1.000000000000000000 ) ) ;
#6325=DIRECTION ( 'NONE',  ( -0.000000000000000000, 1.000000000000000000, -0.000000000000000000 ) ) ;
#6338=ORIENTED_EDGE ( 'NONE', *, *, #6125, .F. ) ;
#6339=CARTESIAN_POINT ( 'NONE',  ( -5.562309845534701758, 60.99999999999999289, 37.56426808735052703 ) ) ;
#6344=CARTESIAN_POINT ( 'NONE',  ( 5.562309845534588959, 69.99999999999998579, -30.56426808735054479 ) ) ;
#6346=CIRCLE ( 'NONE', #3674, 3.000000000000002665 ) ;
#6354=DIRECTION ( 'NONE',  ( 0.000000000000000000, 0.000000000000000000, 1.000000000000000000 ) ) ;
#6356=DIRECTION ( 'NONE',  ( -0.000000000000000000, -1.000000000000000000, -0.000000000000000000 ) ) ;
#6373=PLANE ( 'NONE',  #3619 ) ;
#6375=CARTESIAN_POINT ( 'NONE',  ( 0.000000000000000000, 58.99999999999999289, 0.000000000000000000 ) ) ;
#6376=EDGE_LOOP ( 'NONE', ( #2014, #1815, #1559, #856 ) ) ;
#6377=CYLINDRICAL_SURFACE ( 'NONE', #5911, 38.00000000000000711 ) ;
#6394=CARTESIAN_POINT ( 'NONE',  ( 33.06426808735054124, 69.99999999999998579, 5.562309845534586294 ) ) ;
#6409=CIRCLE ( 'NONE', #9422, 2.500000000000002220 ) ;
#6419=ADVANCED_FACE ( 'NONE', ( #1889 ), #433, .F. ) ;
#6421=EDGE_CURVE ( 'NONE', #6767, #3486, #1200, .T. ) ;
#6435=ORIENTED_EDGE ( 'NONE', *, *, #5344, .T. ) ;
#6442=ORIENTED_EDGE ( 'NONE', *, *, #411, .F. ) ;
#6444=CARTESIAN_POINT ( 'NONE',  ( -5.562309845534584518, 69.99999999999998579, 33.06426808735054124 ) ) ;
#6448=AXIS2_PLACEMENT_3D ( 'NONE', #4220, #6611, #7261 ) ;
#6452=AXIS2_PLACEMENT_3D ( 'NONE', #4386, #3587, #9610 ) ;
#6453=DIRECTION ( 'NONE',  ( 0.000000000000000000, 0.000000000000000000, 1.000000000000000000 ) ) ;
#6468=VERTEX_POINT ( 'NONE', #2671 ) ;
#6471=ORIENTED_EDGE ( 'NONE', *, *, #2617, .F. ) ;
#6472=ADVANCED_FACE ( 'NONE', ( #3471 ), #6473, .F. ) ;
#6473=CYLINDRICAL_SURFACE ( 'NONE', #1353, 1.500000000000001332 ) ;
#6476=DIRECTION ( 'NONE',  ( 0.000000000000000000, -1.000000000000000000, 0.000000000000000000 ) ) ;
#6487=CARTESIAN_POINT ( 'NONE',  ( 0.000000000000000000, 58.99999999999999289, -40.00000000000000711 ) ) ;
#6490=EDGE_CURVE ( 'NONE', #1519, #2516, #6542, .T. ) ;
#6493=VECTOR ( 'NONE', #1640, 1000.000000000000000 ) ;
#6494=EDGE_LOOP ( 'NONE', ( #4996, #4244, #4730, #9595 ) ) ;
#6501=CIRCLE ( 'NONE', #673, 27.99999999999999289 ) ;
#6507=CARTESIAN_POINT ( 'NONE',  ( -33.06426808735054124, 61.99999999999999289, -5.562309845534586294 ) ) ;
#6510=DIRECTION ( 'NONE',  ( 0.000000000000000000, -0.000000000000000000, 1.000000000000000000 ) ) ;
#6526=CARTESIAN_POINT ( 'NONE',  ( 0.000000000000000000, 61.99999999999999289, 0.000000000000000000 ) ) ;
#6529=EDGE_LOOP ( 'NONE', ( #2756, #3695, #8537, #3379, #256 ) ) ;
#6538=LINE ( 'NONE', #537, #8373 ) ;
#6540=CIRCLE ( 'NONE', #2275, 4.500000000000004441 ) ;
#6542=CIRCLE ( 'NONE', #8457, 4.500000000000004441 ) ;
#6545=EDGE_CURVE ( 'NONE', #3486, #3340, #3881, .T. ) ;
#6550=CIRCLE ( 'NONE', #7177, 37.00000000000000711 ) ;
#6556=VECTOR ( 'NONE', #5451, 1000.000000000000000 ) ;
#6557=DIRECTION ( 'NONE',  ( 0.000000000000000000, 1.000000000000000000, 0.000000000000000000 ) ) ;
#6562=CARTESIAN_POINT ( 'NONE',  ( -5.562309845534584518, 59.99999999999999289, 33.06426808735054124 ) ) ;
#6565=CIRCLE ( 'NONE', #4845, 2.500000000000002220 ) ;
#6580=ORIENTED_EDGE ( 'NONE', *, *, #2017, .T. ) ;
#6582=DIRECTION ( 'NONE',  ( 0.000000000000000000, 1.000000000000000000, 0.000000000000000000 ) ) ;
#6583=ORIENTED_EDGE ( 'NONE', *, *, #3112, .F. ) ;
#6590=ORIENTED_EDGE ( 'NONE', *, *, #7387, .F. ) ;
#6603=ORIENTED_EDGE ( 'NONE', *, *, #8179, .T. ) ;
#6607=CIRCLE ( 'NONE', #5973, 4.500000000000005329 ) ;
#6608=DIRECTION ( 'NONE',  ( 0.000000000000000000, -0.000000000000000000, 1.000000000000000000 ) ) ;
#6609=ORIENTED_EDGE ( 'NONE', *, *, #5704, .T. ) ;
#6610=ADVANCED_FACE ( 'NONE', ( #5011 ), #2778, .F. ) ;
#6611=DIRECTION ( 'NONE',  ( 0.000000000000000000, 1.000000000000000000, 0.000000000000000000 ) ) ;
#6615=ORIENTED_EDGE ( 'NONE', *, *, #6001, .F. ) ;
#6619=CIRCLE ( 'NONE', #1269, 27.99999999999999289 ) ;
#6622=CARTESIAN_POINT ( 'NONE',  ( -33.06426808735054124, 69.99999999999998579, -5.562309845534581854 ) ) ;
#6624=CARTESIAN_POINT ( 'NONE',  ( -28.87459861216645862, 60.99999999999999289, -15.97678174684361707 ) ) ;
#6625=ORIENTED_EDGE ( 'NONE', *, *, #8287, .T. ) ;
#6636=CARTESIAN_POINT ( 'NONE',  ( 0.000000000000000000, 61.99999999999999289, 0.000000000000000000 ) ) ;
#6642=AXIS2_PLACEMENT_3D ( 'NONE', #7109, #1782, #6320 ) ;
#6644=DIRECTION ( 'NONE',  ( -0.000000000000000000, -1.000000000000000000, -0.000000000000000000 ) ) ;
#6645=VERTEX_POINT ( 'NONE', #1444 ) ;
#6650=ORIENTED_EDGE ( 'NONE', *, *, #4145, .F. ) ;
#6654=AXIS2_PLACEMENT_3D ( 'NONE', #4049, #5572, #5526 ) ;
#6659=EDGE_CURVE ( 'NONE', #7105, #2210, #258, .T. ) ;
#6668=DIRECTION ( 'NONE',  ( 0.000000000000000000, 0.000000000000000000, 1.000000000000000000 ) ) ;
#6681=CIRCLE ( 'NONE', #3537, 1.500000000000001332 ) ;
#6688=CIRCLE ( 'NONE', #8595, 1.500000000000001332 ) ;
#6692=FACE_BOUND ( 'NONE', #922, .T. ) ;
#6700=EDGE_LOOP ( 'NONE', ( #4123, #9517, #2165, #4828 ) ) ;
#6702=AXIS2_PLACEMENT_3D ( 'NONE', #567, #8901, #707 ) ;
#6704=VERTEX_POINT ( 'NONE', #8808 ) ;
#6712=ORIENTED_EDGE ( 'NONE', *, *, #3282, .F. ) ;
#6727=CARTESIAN_POINT ( 'NONE',  ( 0.000000000000000000, 59.99999999999999289, 0.000000000000000000 ) ) ;
#6730=EDGE_CURVE ( 'NONE', #7154, #6767, #3921, .T. ) ;
#6752=DIRECTION ( 'NONE',  ( -0.000000000000000000, 1.000000000000000000, -0.000000000000000000 ) ) ;
#6758=VECTOR ( 'NONE', #946, 1000.000000000000000 ) ;
#6767=VERTEX_POINT ( 'NONE', #807 ) ;
#6768=EDGE_CURVE ( 'NONE', #1665, #7105, #6022, .T. ) ;
#6772=ADVANCED_FACE ( 'NONE', ( #6816 ), #860, .T. ) ;
#6774=AXIS2_PLACEMENT_3D ( 'NONE', #7788, #9469, #4041 ) ;
#6780=EDGE_CURVE ( 'NONE', #2072, #7884, #1615, .T. ) ;
#6784=CARTESIAN_POINT ( 'NONE',  ( 5.562309845534588959, 60.99999999999999289, -33.06426808735054124 ) ) ;
#6786=DIRECTION ( 'NONE',  ( 0.000000000000000000, 1.000000000000000000, 0.000000000000000000 ) ) ;
#6791=EDGE_CURVE ( 'NONE', #1432, #5694, #4620, .T. ) ;
#6794=DIRECTION ( 'NONE',  ( 0.000000000000000000, 0.000000000000000000, -1.000000000000000000 ) ) ;
#6797=DIRECTION ( 'NONE',  ( -0.000000000000000000, -1.000000000000000000, -0.000000000000000000 ) ) ;
#6802=APPLICATION_CONTEXT ( 'automotive_design' ) ;
#6803=DIRECTION ( 'NONE',  ( -0.000000000000000000, 1.000000000000000000, -0.000000000000000000 ) ) ;
#6814=ORIENTED_EDGE ( 'NONE', *, *, #9268, .T. ) ;
#6816=FACE_OUTER_BOUND ( 'NONE', #7421, .T. ) ;
#6824=ORIENTED_EDGE ( 'NONE', *, *, #2500, .F. ) ;
#6830=FACE_OUTER_BOUND ( 'NONE', #6162, .T. ) ;
#6833=CARTESIAN_POINT ( 'NONE',  ( 34.07933880998927378, 60.99999999999999289, -5.371095444502794081 ) ) ;
#6852=CARTESIAN_POINT ( 'NONE',  ( -28.87459861216645862, 61.99999999999999289, -15.97678174684361707 ) ) ;
#6853=CARTESIAN_POINT ( 'NONE',  ( 3.517955418139624424, 61.99189485091271479, -37.07865250164482518 ) ) ;
#6863=ORIENTED_EDGE ( 'NONE', *, *, #7582, .T. ) ;
#6867=AXIS2_PLACEMENT_3D ( 'NONE', #1479, #752, #9145 ) ;
#6868=AXIS2_PLACEMENT_3D ( 'NONE', #4471, #2727, #9555 ) ;
#6871=AXIS2_PLACEMENT_3D ( 'NONE', #8536, #1764, #6354 ) ;
#6872=ORIENTED_EDGE ( 'NONE', *, *, #4694, .F. ) ;
#6879=DIRECTION ( 'NONE',  ( 0.000000000000000000, -1.000000000000000000, 0.000000000000000000 ) ) ;
#6882=DIRECTION ( 'NONE',  ( 0.000000000000000000, 0.000000000000000000, 1.000000000000000000 ) ) ;
#6890=DIRECTION ( 'NONE',  ( 0.000000000000000000, 0.000000000000000000, 1.000000000000000000 ) ) ;
#6894=CARTESIAN_POINT ( 'NONE',  ( 37.52916669695763119, 61.87792984901915361, 4.938418073206593206 ) ) ;
#6901=ADVANCED_BREP_SHAPE_REPRESENTATION ( '', ( #9444, #6314 ), #3968 ) ;
#6903=ORIENTED_EDGE ( 'NONE', *, *, #7366, .T. ) ;
#6909=ORIENTED_EDGE ( 'NONE', *, *, #6001, .T. ) ;
#6914=DIRECTION ( 'NONE',  ( 0.000000000000000000, 1.000000000000000000, 0.000000000000000000 ) ) ;
#6923=VECTOR ( 'NONE', #6752, 1000.000000000000000 ) ;
#6927=CARTESIAN_POINT ( 'NONE',  ( -33.06426808735054124, 60.99999999999999289, -5.562309845534586294 ) ) ;
#6934=CARTESIAN_POINT ( 'NONE',  ( 2.568784777805632302, 60.99999999999999289, 16.29881421347313974 ) ) ;
#6941=DIRECTION ( 'NONE',  ( -0.000000000000000000, 1.000000000000000000, -0.000000000000000000 ) ) ;
#6942=CARTESIAN_POINT ( 'NONE',  ( 37.42097066196858179, 61.92370482830305889, 4.403127714044224206 ) ) ;
#6943=ORIENTED_EDGE ( 'NONE', *, *, #4021, .T. ) ;
#6944=EDGE_CURVE ( 'NONE', #849, #7361, #9023, .T. ) ;
#6950=DIRECTION ( 'NONE',  ( 0.000000000000000000, 0.000000000000000000, -1.000000000000000000 ) ) ;
#6952=LINE ( 'NONE', #126, #6758 ) ;
#6955=AXIS2_PLACEMENT_3D ( 'NONE', #9129, #6786, #1568 ) ;
#6964=ADVANCED_FACE ( 'NONE', ( #8558 ), #2656, .F. ) ;
#6965=EDGE_LOOP ( 'NONE', ( #8564, #3918 ) ) ;
#6968=DIRECTION ( 'NONE',  ( -0.000000000000000000, 1.000000000000000000, 0.000000000000000000 ) ) ;
#6978=DIRECTION ( 'NONE',  ( 0.000000000000000000, 0.000000000000000000, 1.000000000000000000 ) ) ;
#6990=ORIENTED_EDGE ( 'NONE', *, *, #2601, .T. ) ;
#6992=LINE ( 'NONE', #259, #4302 ) ;
#7003=DIRECTION ( 'NONE',  ( -0.000000000000000000, 1.000000000000000000, -0.000000000000000000 ) ) ;
#7014=VERTEX_POINT ( 'NONE', #5827 ) ;
#7016=CYLINDRICAL_SURFACE ( 'NONE', #9084, 27.99999999999999289 ) ;
#7019=AXIS2_PLACEMENT_3D ( 'NONE', #8331, #1369, #4390 ) ;
#7026=DIRECTION ( 'NONE',  ( -0.000000000000000000, 1.000000000000000000, -0.000000000000000000 ) ) ;
#7033=VECTOR ( 'NONE', #1638, 1000.000000000000000 ) ;
#7037=CARTESIAN_POINT ( 'NONE',  ( 0.000000000000000000, 60.99999999999999289, 0.000000000000000000 ) ) ;
#7046=CARTESIAN_POINT ( 'NONE',  ( -36.86535760663189620, 61.99999999999999289, -3.153634179030289530 ) ) ;
#7051=CARTESIAN_POINT ( 'NONE',  ( 15.97678174684330799, 60.99999999999999289, -28.87459861216662205 ) ) ;
#7052=VERTEX_POINT ( 'NONE', #9675 ) ;
#7059=VERTEX_POINT ( 'NONE', #8797 ) ;
#7061=EDGE_LOOP ( 'NONE', ( #4804, #6990, #7827, #7783 ) ) ;
#7064=ORIENTED_EDGE ( 'NONE', *, *, #5282, .F. ) ;
#7077=DIRECTION ( 'NONE',  ( 0.000000000000000000, 1.000000000000000000, 0.000000000000000000 ) ) ;
#7080=CARTESIAN_POINT ( 'NONE',  ( -30.18708036726492594, 60.99999999999999289, -16.70299909897287094 ) ) ;
#7090=VECTOR ( 'NONE', #304, 1000.000000000000000 ) ;
#7098=LINE ( 'NONE', #1961, #3535 ) ;
#7101=CARTESIAN_POINT ( 'NONE',  ( -36.80315167070719440, 61.92350945662830952, -8.081333402833552171 ) ) ;
#7105=VERTEX_POINT ( 'NONE', #9485 ) ;
#7106=DIRECTION ( 'NONE',  ( 0.000000000000000000, 0.000000000000000000, 1.000000000000000000 ) ) ;
#7109=CARTESIAN_POINT ( 'NONE',  ( 33.06426808735054124, 69.99999999999998579, 5.562309845534586294 ) ) ;
#7114=VERTEX_POINT ( 'NONE', #7257 ) ;
#7139=ORIENTED_EDGE ( 'NONE', *, *, #2601, .F. ) ;
#7141=VERTEX_POINT ( 'NONE', #4651 ) ;
#7147=EDGE_CURVE ( 'NONE', #2169, #3433, #9340, .T. ) ;
#7151=CARTESIAN_POINT ( 'NONE',  ( 30.18708036726505028, 61.99999999999999289, 16.70299909897265778 ) ) ;
#7154=VERTEX_POINT ( 'NONE', #9191 ) ;
#7156=ORIENTED_EDGE ( 'NONE', *, *, #3712, .T. ) ;
#7163=( LENGTH_UNIT ( ) NAMED_UNIT ( * ) SI_UNIT ( .MILLI., .METRE. ) );
#7167=CARTESIAN_POINT ( 'NONE',  ( 33.06426808735054124, 59.99999999999999289, 8.062309845534588959 ) ) ;
#7175=CARTESIAN_POINT ( 'NONE',  ( -5.562309845534584518, 69.99999999999998579, 33.06426808735054124 ) ) ;
#7177=AXIS2_PLACEMENT_3D ( 'NONE', #795, #5286, #8301 ) ;
#7179=ORIENTED_EDGE ( 'NONE', *, *, #1609, .T. ) ;
#7180=DIRECTION ( 'NONE',  ( 0.000000000000000000, 1.000000000000000000, 0.000000000000000000 ) ) ;
#7182=EDGE_CURVE ( 'NONE', #5814, #7014, #6174, .T. ) ;
#7183=CIRCLE ( 'NONE', #7019, 2.500000000000002220 ) ;
#7191=AXIS2_PLACEMENT_3D ( 'NONE', #4848, #4750, #6950 ) ;
#7205=EDGE_CURVE ( 'NONE', #1252, #2652, #1766, .T. ) ;
#7206=ORIENTED_EDGE ( 'NONE', *, *, #35, .F. ) ;
#7228=EDGE_LOOP ( 'NONE', ( #2473, #7679, #2668, #377 ) ) ;
#7236=CYLINDRICAL_SURFACE ( 'NONE', #7975, 2.500000000000001332 ) ;
#7240=CYLINDRICAL_SURFACE ( 'NONE', #3743, 34.49999999999998579 ) ;
#7241=DIRECTION ( 'NONE',  ( 0.000000000000000000, 0.000000000000000000, 1.000000000000000000 ) ) ;
#7246=CIRCLE ( 'NONE', #477, 38.00000000000000711 ) ;
#7252=CARTESIAN_POINT ( 'NONE',  ( 0.000000000000000000, 61.99999999999999289, 0.000000000000000000 ) ) ;
#7254=EDGE_CURVE ( 'NONE', #7682, #8580, #362, .T. ) ;
#7256=AXIS2_PLACEMENT_3D ( 'NONE', #4476, #1998, #8868 ) ;
#7257=CARTESIAN_POINT ( 'NONE',  ( -15.25056439471426195, 61.99999999999999289, 27.56211685706803038 ) ) ;
#7258=LINE ( 'NONE', #506, #4043 ) ;
#7259=EDGE_CURVE ( 'NONE', #5164, #8683, #5411, .T. ) ;
#7260=ADVANCED_FACE ( 'NONE', ( #1529 ), #2308, .F. ) ;
#7261=DIRECTION ( 'NONE',  ( 0.000000000000000000, 0.000000000000000000, 1.000000000000000000 ) ) ;
#7264=DIRECTION ( 'NONE',  ( 0.000000000000000000, 0.000000000000000000, 1.000000000000000000 ) ) ;
#7276=CYLINDRICAL_SURFACE ( 'NONE', #8435, 1.500000000000003109 ) ;
#7278=ORIENTED_EDGE ( 'NONE', *, *, #3282, .T. ) ;
#7287=AXIS2_PLACEMENT_3D ( 'NONE', #1630, #1474, #3147 ) ;
#7297=AXIS2_PLACEMENT_3D ( 'NONE', #298, #3247, #203 ) ;
#7298=CARTESIAN_POINT ( 'NONE',  ( -32.59762842694629370, 60.99999999999999289, 5.137569555611143812 ) ) ;
#7300=AXIS2_PLACEMENT_3D ( 'NONE', #1784, #3363, #5643 ) ;
#7302=DIRECTION ( 'NONE',  ( 0.000000000000000000, 0.000000000000000000, -1.000000000000000000 ) ) ;
#7304=CARTESIAN_POINT ( 'NONE',  ( -33.06426808735054124, 60.99999999999999289, -5.562309845534586294 ) ) ;
#7306=VERTEX_POINT ( 'NONE', #7799 ) ;
#7308=DIRECTION ( 'NONE',  ( 0.000000000000000000, 1.000000000000000000, 0.000000000000000000 ) ) ;
#7313=ORIENTED_EDGE ( 'NONE', *, *, #7761, .T. ) ;
#7317=AXIS2_PLACEMENT_3D ( 'NONE', #4096, #340, #3141 ) ;
#7319=VERTEX_POINT ( 'NONE', #1866 ) ;
#7323=AXIS2_PLACEMENT_3D ( 'NONE', #7037, #293, #838 ) ;
#7328=VERTEX_POINT ( 'NONE', #4102 ) ;
#7334=AXIS2_PLACEMENT_3D ( 'NONE', #8679, #3440, #2737 ) ;
#7341=CIRCLE ( 'NONE', #1820, 37.00000000000000711 ) ;
#7350=DIRECTION ( 'NONE',  ( 0.000000000000000000, 0.000000000000000000, 1.000000000000000000 ) ) ;
#7359=DIRECTION ( 'NONE',  ( 0.000000000000000000, 1.000000000000000000, 0.000000000000000000 ) ) ;
#7360=CARTESIAN_POINT ( 'NONE',  ( -28.87459861216645862, 61.99999999999999289, -15.97678174684361707 ) ) ;
#7361=VERTEX_POINT ( 'NONE', #4795 ) ;
#7366=EDGE_CURVE ( 'NONE', #9614, #7306, #8402, .T. ) ;
#7374=FACE_BOUND ( 'NONE', #5660, .T. ) ;
#7387=EDGE_CURVE ( 'NONE', #6468, #1101, #6013, .T. ) ;
#7392=ORIENTED_EDGE ( 'NONE', *, *, #2534, .F. ) ;
#7393=CARTESIAN_POINT ( 'NONE',  ( -6.235648121649205677, 61.81426382726520075, 37.52627707316312922 ) ) ;
#7402=EDGE_CURVE ( 'NONE', #8252, #2652, #6992, .T. ) ;
#7405=DIRECTION ( 'NONE',  ( -0.000000000000000000, -1.000000000000000000, -0.000000000000000000 ) ) ;
#7411=CIRCLE ( 'NONE', #8829, 1.500000000000001332 ) ;
#7421=EDGE_LOOP ( 'NONE', ( #8839, #3509, #3057, #6625, #286 ) ) ;
#7429=AXIS2_PLACEMENT_3D ( 'NONE', #1711, #9228, #9180 ) ;
#7430=ORIENTED_EDGE ( 'NONE', *, *, #1241, .T. ) ;
#7431=FACE_OUTER_BOUND ( 'NONE', #2655, .T. ) ;
#7439=VERTEX_POINT ( 'NONE', #1767 ) ;
#7446=EDGE_CURVE ( 'NONE', #5699, #7580, #7932, .T. ) ;
#7447=CARTESIAN_POINT ( 'NONE',  ( 5.562309845534932684, 61.83753588906734677, -37.56426808735049150 ) ) ;
#7448=AXIS2_PLACEMENT_3D ( 'NONE', #2355, #8345, #4702 ) ;
#7460=DIRECTION ( 'NONE',  ( 0.000000000000000000, 1.000000000000000000, 0.000000000000000000 ) ) ;
#7468=ORIENTED_EDGE ( 'NONE', *, *, #3765, .F. ) ;
#7474=CARTESIAN_POINT ( 'NONE',  ( 0.000000000000000000, 59.99999999999999289, 0.000000000000000000 ) ) ;
#7476=ORIENTED_EDGE ( 'NONE', *, *, #8375, .T. ) ;
#7485=ADVANCED_FACE ( 'NONE', ( #769 ), #4478, .T. ) ;
#7492=EDGE_CURVE ( 'NONE', #2210, #7105, #6501, .T. ) ;
#7503=ORIENTED_EDGE ( 'NONE', *, *, #5657, .T. ) ;
#7505=DIRECTION ( 'NONE',  ( 0.000000000000000000, 1.000000000000000000, 0.000000000000000000 ) ) ;
#7509=CARTESIAN_POINT ( 'NONE',  ( -33.06426808735054124, 60.99999999999999289, -5.562309845534586294 ) ) ;
#7510=AXIS2_PLACEMENT_3D ( 'NONE', #857, #802, #3813 ) ;
#7516=ORIENTED_EDGE ( 'NONE', *, *, #1515, .T. ) ;
#7517=CARTESIAN_POINT ( 'NONE',  ( 35.86802812777743554, 61.99999999999999289, 9.082100980773358145 ) ) ;
#7522=ORIENTED_EDGE ( 'NONE', *, *, #9032, .F. ) ;
#7526=CARTESIAN_POINT ( 'NONE',  ( -5.137569555611031014, 60.99999999999999289, -32.59762842694632212 ) ) ;
#7535=UNCERTAINTY_MEASURE_WITH_UNIT (LENGTH_MEASURE( 1.000000000000000082E-05 ), #2749, 'distance_accuracy_value', 'NONE');
#7546=CARTESIAN_POINT ( 'NONE',  ( -9.082100980773482490, 61.99999999999999289, 35.86802812777740002 ) ) ;
#7548=CARTESIAN_POINT ( 'NONE',  ( -15.97678174684350871, 61.99999999999999289, 30.37459861216651191 ) ) ;
#7555=CARTESIAN_POINT ( 'NONE',  ( 0.000000000000000000, 59.99999999999999289, -37.00000000000000711 ) ) ;
#7571=ORIENTED_EDGE ( 'NONE', *, *, #4929, .F. ) ;
#7573=AXIS2_PLACEMENT_3D ( 'NONE', #1879, #4903, #4169 ) ;
#7575=CARTESIAN_POINT ( 'NONE',  ( -3.517955418139367740, 61.99189485091269347, 37.07865250164484650 ) ) ;
#7577=ORIENTED_EDGE ( 'NONE', *, *, #5319, .T. ) ;
#7579=ORIENTED_EDGE ( 'NONE', *, *, #1609, .F. ) ;
#7580=VERTEX_POINT ( 'NONE', #4294 ) ;
#7582=EDGE_CURVE ( 'NONE', #4514, #9543, #6183, .T. ) ;
#7583=EDGE_CURVE ( 'NONE', #7681, #3498, #1610, .T. ) ;
#7590=VERTEX_POINT ( 'NONE', #1650 ) ;
#7591=CARTESIAN_POINT ( 'NONE',  ( -5.902069945235074222, 61.82045560759793545, 37.56426808735054124 ) ) ;
#7593=CARTESIAN_POINT ( 'NONE',  ( 0.000000000000000000, 58.99999999999999289, 0.000000000000000000 ) ) ;
#7598=EDGE_LOOP ( 'NONE', ( #4683, #4147 ) ) ;
#7603=ORIENTED_EDGE ( 'NONE', *, *, #4862, .F. ) ;
#7623=AXIS2_PLACEMENT_3D ( 'NONE', #8393, #692, #896 ) ;
#7630=ORIENTED_EDGE ( 'NONE', *, *, #889, .F. ) ;
#7631=DIRECTION ( 'NONE',  ( 0.000000000000000000, 0.000000000000000000, 1.000000000000000000 ) ) ;
#7637=CYLINDRICAL_SURFACE ( 'NONE', #3406, 34.50000000000000000 ) ;
#7640=AXIS2_PLACEMENT_3D ( 'NONE', #6784, #1458, #731 ) ;
#7647=CARTESIAN_POINT ( 'NONE',  ( 0.000000000000000000, 52.29648987751954792, 0.000000000000000000 ) ) ;
#7649=EDGE_CURVE ( 'NONE', #1665, #6026, #5088, .T. ) ;
#7652=CARTESIAN_POINT ( 'NONE',  ( 37.08058572124223673, 61.87769929713620343, 7.610216775991024640 ) ) ;
#7655=VECTOR ( 'NONE', #2445, 1000.000000000000000 ) ;
#7657=LINE ( 'NONE', #901, #1348 ) ;
#7669=ORIENTED_EDGE ( 'NONE', *, *, #3586, .T. ) ;
#7673=AXIS2_PLACEMENT_3D ( 'NONE', #6118, #904, #162 ) ;
#7675=ADVANCED_FACE ( 'NONE', ( #4678 ), #5511, .F. ) ;
#7679=ORIENTED_EDGE ( 'NONE', *, *, #3712, .F. ) ;
#7680=CYLINDRICAL_SURFACE ( 'NONE', #1350, 4.500000000000003553 ) ;
#7681=VERTEX_POINT ( 'NONE', #3224 ) ;
#7682=VERTEX_POINT ( 'NONE', #5363 ) ;
#7691=CARTESIAN_POINT ( 'NONE',  ( -33.06426808735054124, 59.99999999999999289, -5.562309845534581854 ) ) ;
#7693=CYLINDRICAL_SURFACE ( 'NONE', #2521, 40.00000000000000711 ) ;
#7695=ORIENTED_EDGE ( 'NONE', *, *, #7791, .F. ) ;
#7697=EDGE_CURVE ( 'NONE', #7306, #3340, #8519, .T. ) ;
#7701=LINE ( 'NONE', #9324, #1773 ) ;
#7702=CARTESIAN_POINT ( 'NONE',  ( 36.08344047792740383, 62.00000000000266454, 8.910509964045653319 ) ) ;
#7709=CARTESIAN_POINT ( 'NONE',  ( 32.59762842694625817, 60.99999999999999289, -5.137569555611371186 ) ) ;
#7713=DIRECTION ( 'NONE',  ( 0.000000000000000000, 1.000000000000000000, 0.000000000000000000 ) ) ;
#7730=CARTESIAN_POINT ( 'NONE',  ( -16.29881421347314685, 60.99999999999999289, 2.568784777805571906 ) ) ;
#7731=DIRECTION ( 'NONE',  ( -0.000000000000000000, 1.000000000000000000, -0.000000000000000000 ) ) ;
#7732=ORIENTED_EDGE ( 'NONE', *, *, #4456, .T. ) ;
#7735=CARTESIAN_POINT ( 'NONE',  ( 33.06426808735054124, 60.99999999999999289, 5.562309845534586294 ) ) ;
#7745=FACE_OUTER_BOUND ( 'NONE', #4526, .T. ) ;
#7746=CARTESIAN_POINT ( 'NONE',  ( 36.86535760663189620, 61.99999999999999289, 3.153634179030289530 ) ) ;
#7751=CARTESIAN_POINT ( 'NONE',  ( 33.06426808735054124, 60.99999999999999289, 3.062309845534584074 ) ) ;
#7756=ORIENTED_EDGE ( 'NONE', *, *, #4145, .T. ) ;
#7761=EDGE_CURVE ( 'NONE', #2719, #1252, #372, .T. ) ;
#7764=FACE_OUTER_BOUND ( 'NONE', #6529, .T. ) ;
#7767=VERTEX_POINT ( 'NONE', #1062 ) ;
#7769=ADVANCED_FACE ( 'NONE', ( #8716 ), #2522, .F. ) ;
#7780=AXIS2_PLACEMENT_3D ( 'NONE', #7175, #6476, #3374 ) ;
#7783=ORIENTED_EDGE ( 'NONE', *, *, #7182, .F. ) ;
#7788=CARTESIAN_POINT ( 'NONE',  ( -5.562309845534701758, 60.99999999999999289, 33.06426808735052703 ) ) ;
#7791=EDGE_CURVE ( 'NONE', #5322, #8683, #6346, .T. ) ;
#7792=CIRCLE ( 'NONE', #1955, 4.500000000000005329 ) ;
#7799=CARTESIAN_POINT ( 'NONE',  ( 16.70299909897254409, 60.99999999999999289, -30.18708036726510002 ) ) ;
#7803=CARTESIAN_POINT ( 'NONE',  ( 5.562309845534933572, 60.99999999999999289, -37.56426808735049150 ) ) ;
#7811=VERTEX_POINT ( 'NONE', #8568 ) ;
#7813=AXIS2_PLACEMENT_3D ( 'NONE', #8950, #4408, #7264 ) ;
#7826=AXIS2_PLACEMENT_3D ( 'NONE', #353, #2461, #5579 ) ;
#7827=ORIENTED_EDGE ( 'NONE', *, *, #4565, .T. ) ;
#7851=EDGE_LOOP ( 'NONE', ( #2400, #6299, #1646, #32 ) ) ;
#7858=VERTEX_POINT ( 'NONE', #376 ) ;
#7865=ORIENTED_EDGE ( 'NONE', *, *, #249, .F. ) ;
#7875=FACE_OUTER_BOUND ( 'NONE', #7228, .T. ) ;
#7882=ORIENTED_EDGE ( 'NONE', *, *, #7259, .F. ) ;
#7884=VERTEX_POINT ( 'NONE', #3575 ) ;
#7904=CIRCLE ( 'NONE', #1899, 34.50000000000000000 ) ;
#7908=LINE ( 'NONE', #1087, #1825 ) ;
#7909=ORIENTED_EDGE ( 'NONE', *, *, #7205, .F. ) ;
#7911=CARTESIAN_POINT ( 'NONE',  ( 33.06426808735054124, 59.99999999999999289, 5.562309845534586294 ) ) ;
#7918=AXIS2_PLACEMENT_3D ( 'NONE', #7735, #4781, #6287 ) ;
#7920=DIRECTION ( 'NONE',  ( 0.000000000000000000, 0.000000000000000000, -1.000000000000000000 ) ) ;
#7932=CIRCLE ( 'NONE', #8241, 38.00000000000000711 ) ;
#7935=DIRECTION ( 'NONE',  ( 0.000000000000000000, 0.000000000000000000, 1.000000000000000000 ) ) ;
#7954=AXIS2_PLACEMENT_3D ( 'NONE', #3333, #3984, #2481 ) ;
#7965=EDGE_LOOP ( 'NONE', ( #1028, #5241, #8663, #6282, #7064 ) ) ;
#7966=CARTESIAN_POINT ( 'NONE',  ( -35.86802812777743554, 61.99999999999999289, -9.082100980773358145 ) ) ;
#7969=ORIENTED_EDGE ( 'NONE', *, *, #3765, .T. ) ;
#7975=AXIS2_PLACEMENT_3D ( 'NONE', #1999, #385, #4141 ) ;
#7980=CARTESIAN_POINT ( 'NONE',  ( 0.000000000000000000, 61.99999999999999289, 0.000000000000000000 ) ) ;
#7990=MECHANICAL_DESIGN_GEOMETRIC_PRESENTATION_REPRESENTATION('',(#3416),#8779);
#7992=CARTESIAN_POINT ( 'NONE',  ( 0.000000000000000000, 61.99999999999999289, 0.000000000000000000 ) ) ;
#8021=CARTESIAN_POINT ( 'NONE',  ( 4.531193156845207581E-15, 58.99999999999999289, 37.00000000000000711 ) ) ;
#8031=DIRECTION ( 'NONE',  ( -0.000000000000000000, -1.000000000000000000, -0.000000000000000000 ) ) ;
#8035=CARTESIAN_POINT ( 'NONE',  ( 5.562309845534932684, 60.99999999999999289, -33.06426808735049150 ) ) ;
#8049=CIRCLE ( 'NONE', #3315, 34.50000000000000000 ) ;
#8058=ORIENTED_EDGE ( 'NONE', *, *, #8490, .F. ) ;
#8072=CARTESIAN_POINT ( 'NONE',  ( 4.592425496802575156E-15, 59.99999999999999289, 37.00000000000000711 ) ) ;
#8080=FACE_OUTER_BOUND ( 'NONE', #3600, .T. ) ;
#8087=DIRECTION ( 'NONE',  ( -0.000000000000000000, 1.000000000000000000, -0.000000000000000000 ) ) ;
#8091=ADVANCED_FACE ( 'NONE', ( #7764 ), #1641, .F. ) ;
#8094=FACE_OUTER_BOUND ( 'NONE', #6376, .T. ) ;
#8095=ORIENTED_EDGE ( 'NONE', *, *, #6421, .F. ) ;
#8103=EDGE_CURVE ( 'NONE', #7052, #7811, #5103, .T. ) ;
#8108=ORIENTED_EDGE ( 'NONE', *, *, #3652, .T. ) ;
#8117=AXIS2_PLACEMENT_3D ( 'NONE', #4398, #7405, #4941 ) ;
#8122=VERTEX_POINT ( 'NONE', #1598 ) ;
#8128=ADVANCED_FACE ( 'NONE', ( #175 ), #9157, .F. ) ;
#8131=AXIS2_PLACEMENT_3D ( 'NONE', #4258, #7308, #6608 ) ;
#8135=DIRECTION ( 'NONE',  ( 0.000000000000000000, 1.000000000000000000, 0.000000000000000000 ) ) ;
#8151=ORIENTED_EDGE ( 'NONE', *, *, #6730, .T. ) ;
#8162=EDGE_LOOP ( 'NONE', ( #9062, #9455, #6284, #2626 ) ) ;
#8164=EDGE_LOOP ( 'NONE', ( #1368, #4325, #15, #763 ) ) ;
#8169=CARTESIAN_POINT ( 'NONE',  ( 0.000000000000000000, 0.000000000000000000, 0.000000000000000000 ) ) ;
#8170=ORIENTED_EDGE ( 'NONE', *, *, #4387, .T. ) ;
#8174=CARTESIAN_POINT ( 'NONE',  ( -32.59762842694629370, 60.99999999999999289, 5.137569555611143812 ) ) ;
#8179=EDGE_CURVE ( 'NONE', #344, #8621, #6029, .T. ) ;
#8187=CARTESIAN_POINT ( 'NONE',  ( 34.07933880998927378, 60.99999999999999289, -5.371095444502794081 ) ) ;
#8192=FACE_OUTER_BOUND ( 'NONE', #7851, .T. ) ;
#8197=CARTESIAN_POINT ( 'NONE',  ( 5.562309845534932684, 61.99999999999999289, -33.06426808735049150 ) ) ;
#8204=VERTEX_POINT ( 'NONE', #6271 ) ;
#8227=CARTESIAN_POINT ( 'NONE',  ( -5.562309845534584518, 60.99999999999999289, 33.06426808735054124 ) ) ;
#8231=LINE ( 'NONE', #5181, #4658 ) ;
#8233=AXIS2_PLACEMENT_3D ( 'NONE', #3869, #9205, #9156 ) ;
#8241=AXIS2_PLACEMENT_3D ( 'NONE', #6306, #1035, #4054 ) ;
#8252=VERTEX_POINT ( 'NONE', #4900 ) ;
#8255=LINE ( 'NONE', #6075, #4819 ) ;
#8273=CIRCLE ( 'NONE', #7640, 2.499999999999998668 ) ;
#8277=ORIENTED_EDGE ( 'NONE', *, *, #51, .F. ) ;
#8280=CARTESIAN_POINT ( 'NONE',  ( 0.000000000000000000, 61.99999999999999289, 0.000000000000000000 ) ) ;
#8287=EDGE_CURVE ( 'NONE', #326, #6704, #5909, .T. ) ;
#8290=ORIENTED_EDGE ( 'NONE', *, *, #7791, .T. ) ;
#8293=AXIS2_PLACEMENT_3D ( 'NONE', #7992, #4287, #491 ) ;
#8301=DIRECTION ( 'NONE',  ( 0.000000000000000000, 0.000000000000000000, -1.000000000000000000 ) ) ;
#8305=ORIENTED_EDGE ( 'NONE', *, *, #2240, .T. ) ;
#8327=DIRECTION ( 'NONE',  ( 0.000000000000000000, 0.000000000000000000, -1.000000000000000000 ) ) ;
#8331=CARTESIAN_POINT ( 'NONE',  ( 33.06426808735054124, 60.99999999999999289, 5.562309845534586294 ) ) ;
#8338=FACE_OUTER_BOUND ( 'NONE', #449, .T. ) ;
#8342=CARTESIAN_POINT ( 'NONE',  ( 31.11591804390324612, 61.99999999999999289, -4.904043666719942074 ) ) ;
#8345=DIRECTION ( 'NONE',  ( 0.000000000000000000, 1.000000000000000000, 0.000000000000000000 ) ) ;
#8363=DIRECTION ( 'NONE',  ( 0.000000000000000000, 0.000000000000000000, 1.000000000000000000 ) ) ;
#8366=AXIS2_PLACEMENT_3D ( 'NONE', #6927, #3982, #7631 ) ;
#8373=VECTOR ( 'NONE', #8818, 1000.000000000000000 ) ;
#8375=EDGE_CURVE ( 'NONE', #2516, #4765, #4669, .T. ) ;
#8379=CARTESIAN_POINT ( 'NONE',  ( 0.000000000000000000, 61.99999999999999289, 0.000000000000000000 ) ) ;
#8393=CARTESIAN_POINT ( 'NONE',  ( 5.562309845534588959, 60.99999999999999289, -33.06426808735054124 ) ) ;
#8396=ORIENTED_EDGE ( 'NONE', *, *, #7182, .T. ) ;
#8402=CIRCLE ( 'NONE', #8872, 34.49999999999999289 ) ;
#8411=CARTESIAN_POINT ( 'NONE',  ( -4.104483837743832630, 61.95009619975343185, 37.32687308866060505 ) ) ;
#8413=ADVANCED_FACE ( 'NONE', ( #2855 ), #5787, .T. ) ;
#8414=VERTEX_POINT ( 'NONE', #5962 ) ;
#8435=AXIS2_PLACEMENT_3D ( 'NONE', #6624, #8961, #4277 ) ;
#8437=AXIS2_PLACEMENT_3D ( 'NONE', #7647, #4544, #3642 ) ;
#8443=DIRECTION ( 'NONE',  ( 0.000000000000000000, 0.000000000000000000, 1.000000000000000000 ) ) ;
#8445=AXIS2_PLACEMENT_3D ( 'NONE', #7252, #9530, #2103 ) ;
#8446=AXIS2_PLACEMENT_3D ( 'NONE', #8174, #1405, #4332 ) ;
#8450=AXIS2_PLACEMENT_3D ( 'NONE', #7709, #6803, #4653 ) ;
#8451=VECTOR ( 'NONE', #3859, 1000.000000000000000 ) ;
#8452=EDGE_CURVE ( 'NONE', #849, #7052, #5188, .T. ) ;
#8457=AXIS2_PLACEMENT_3D ( 'NONE', #1060, #4128, #9307 ) ;
#8463=CIRCLE ( 'NONE', #7826, 1.500000000000000888 ) ;
#8468=ORIENTED_EDGE ( 'NONE', *, *, #7446, .T. ) ;
#8476=EDGE_CURVE ( 'NONE', #8999, #8611, #7258, .T. ) ;
#8480=ORIENTED_EDGE ( 'NONE', *, *, #1515, .F. ) ;
#8490=EDGE_CURVE ( 'NONE', #5790, #1519, #3209, .T. ) ;
#8492=DIRECTION ( 'NONE',  ( 0.000000000000000000, 0.000000000000000000, 1.000000000000000000 ) ) ;
#8495=CARTESIAN_POINT ( 'NONE',  ( 8.871504613779926274, 62.00000000000265743, -36.13240710991932048 ) ) ;
#8496=CARTESIAN_POINT ( 'NONE',  ( 36.64076086657617282, 61.94822636785970360, 8.307112375470062204 ) ) ;
#8499=CARTESIAN_POINT ( 'NONE',  ( -35.86802812777743554, 61.99999999999999289, -9.082100980773358145 ) ) ;
#8502=EDGE_CURVE ( 'NONE', #2405, #8204, #6550, .T. ) ;
#8504=ORIENTED_EDGE ( 'NONE', *, *, #1947, .T. ) ;
#8505=DIRECTION ( 'NONE',  ( 0.000000000000000000, 0.000000000000000000, 1.000000000000000000 ) ) ;
#8506=DIRECTION ( 'NONE',  ( 0.000000000000000000, 1.000000000000000000, 0.000000000000000000 ) ) ;
#8517=ORIENTED_EDGE ( 'NONE', *, *, #9122, .F. ) ;
#8519=LINE ( 'NONE', #2382, #4631 ) ;
#8521=CIRCLE ( 'NONE', #4419, 2.500000000000002220 ) ;
#8529=LINE ( 'NONE', #6252, #7655 ) ;
#8535=CARTESIAN_POINT ( 'NONE',  ( 7.819489076939989403, 61.89591950820473443, -36.97167050927863130 ) ) ;
#8536=CARTESIAN_POINT ( 'NONE',  ( 0.000000000000000000, 58.99999999999999289, -37.00000000000000711 ) ) ;
#8537=ORIENTED_EDGE ( 'NONE', *, *, #8452, .T. ) ;
#8547=CYLINDRICAL_SURFACE ( 'NONE', #85, 31.49999999999999289 ) ;
#8548=ADVANCED_FACE ( 'NONE', ( #4550 ), #1475, .F. ) ;
#8549=ORIENTED_EDGE ( 'NONE', *, *, #1061, .F. ) ;
#8552=DIRECTION ( 'NONE',  ( -0.000000000000000000, 1.000000000000000000, -0.000000000000000000 ) ) ;
#8556=EDGE_CURVE ( 'NONE', #7590, #1536, #7657, .T. ) ;
#8558=FACE_OUTER_BOUND ( 'NONE', #2274, .T. ) ;
#8564=ORIENTED_EDGE ( 'NONE', *, *, #4694, .T. ) ;
#8568=CARTESIAN_POINT ( 'NONE',  ( -3.153634179030417872, 61.99999999999999289, 36.86535760663188199 ) ) ;
#8580=VERTEX_POINT ( 'NONE', #4703 ) ;
#8584=CARTESIAN_POINT ( 'NONE',  ( 6.890850105526419966, 61.82663791069490600, -37.37679511928140386 ) ) ;
#8595=AXIS2_PLACEMENT_3D ( 'NONE', #7051, #1734, #7106 ) ;
#8610=EDGE_CURVE ( 'NONE', #9714, #8999, #2604, .T. ) ;
#8611=VERTEX_POINT ( 'NONE', #7151 ) ;
#8613=CARTESIAN_POINT ( 'NONE',  ( 3.153634179030674556, 61.99999999999999289, -36.86535760663186068 ) ) ;
#8620=CIRCLE ( 'NONE', #6081, 2.500000000000002220 ) ;
#8621=VERTEX_POINT ( 'NONE', #1726 ) ;
#8622=CIRCLE ( 'NONE', #6868, 37.00000000000000711 ) ;
#8624=DIRECTION ( 'NONE',  ( 0.000000000000000000, 0.000000000000000000, 1.000000000000000000 ) ) ;
#8634=CARTESIAN_POINT ( 'NONE',  ( 5.371095444502685723, 60.99999999999999289, 34.07933880998929510 ) ) ;
#8640=PLANE ( 'NONE',  #4306 ) ;
#8642=EDGE_LOOP ( 'NONE', ( #9109, #8850, #3158, #1531 ) ) ;
#8648=ORIENTED_EDGE ( 'NONE', *, *, #4021, .F. ) ;
#8653=CARTESIAN_POINT ( 'NONE',  ( -5.562309845534701758, 60.99999999999999289, 33.06426808735052703 ) ) ;
#8661=CARTESIAN_POINT ( 'NONE',  ( 0.000000000000000000, 0.000000000000000000, 0.000000000000000000 ) ) ;
#8663=ORIENTED_EDGE ( 'NONE', *, *, #7254, .F. ) ;
#8666=EDGE_CURVE ( 'NONE', #1639, #8204, #5934, .T. ) ;
#8679=CARTESIAN_POINT ( 'NONE',  ( 0.000000000000000000, 61.99999999999999289, 0.000000000000000000 ) ) ;
#8680=AXIS2_PLACEMENT_3D ( 'NONE', #3534, #3390, #8778 ) ;
#8683=VERTEX_POINT ( 'NONE', #6308 ) ;
#8687=PRODUCT_DEFINITION_SHAPE ( 'NONE', 'NONE',  #850 ) ;
#8707=EDGE_LOOP ( 'NONE', ( #6442, #3664 ) ) ;
#8710=FACE_OUTER_BOUND ( 'NONE', #4193, .T. ) ;
#8716=FACE_OUTER_BOUND ( 'NONE', #3644, .T. ) ;
#8724=CARTESIAN_POINT ( 'NONE',  ( 0.000000000000000000, 52.29648987751954792, 0.000000000000000000 ) ) ;
#8729=AXIS2_PLACEMENT_3D ( 'NONE', #3799, #6797, #4494 ) ;
#8734=CARTESIAN_POINT ( 'NONE',  ( 28.87459861216657231, 61.99999999999999289, 15.97678174684340924 ) ) ;
#8736=ORIENTED_EDGE ( 'NONE', *, *, #5211, .T. ) ;
#8738=CARTESIAN_POINT ( 'NONE',  ( 4.531193156845207581E-15, 58.99999999999999289, 37.00000000000000711 ) ) ;
#8739=CARTESIAN_POINT ( 'NONE',  ( 0.000000000000000000, 59.99999999999999289, 0.000000000000000000 ) ) ;
#8743=FACE_BOUND ( 'NONE', #5525, .T. ) ;
#8744=DIRECTION ( 'NONE',  ( 0.000000000000000000, 1.000000000000000000, 0.000000000000000000 ) ) ;
#8757=ORIENTED_EDGE ( 'NONE', *, *, #4032, .T. ) ;
#8765=DIRECTION ( 'NONE',  ( 0.000000000000000000, 1.000000000000000000, 0.000000000000000000 ) ) ;
#8767=CIRCLE ( 'NONE', #8293, 34.50000000000000000 ) ;
#8775=FACE_OUTER_BOUND ( 'NONE', #1063, .T. ) ;
#8777=ADVANCED_FACE ( 'NONE', ( #1019 ), #7637, .F. ) ;
#8778=DIRECTION ( 'NONE',  ( 0.000000000000000000, 0.000000000000000000, 1.000000000000000000 ) ) ;
#8779=( GEOMETRIC_REPRESENTATION_CONTEXT ( 3 ) GLOBAL_UNCERTAINTY_ASSIGNED_CONTEXT ( ( #7535 ) ) GLOBAL_UNIT_ASSIGNED_CONTEXT ( ( #2749, #5770, #2695 ) ) REPRESENTATION_CONTEXT ( 'NONE', 'WORKASPACE' ) );
#8786=DIRECTION ( 'NONE',  ( -1.224646799147349509E-16, 0.000000000000000000, -1.000000000000000000 ) ) ;
#8787=ADVANCED_FACE ( 'NONE', ( #830 ), #3839, .F. ) ;
#8796=EDGE_CURVE ( 'NONE', #1498, #5153, #584, .T. ) ;
#8797=CARTESIAN_POINT ( 'NONE',  ( -15.25056439471426195, 60.99999999999999289, 27.56211685706803038 ) ) ;
#8802=CYLINDRICAL_SURFACE ( 'NONE', #7813, 4.500000000000005329 ) ;
#8808=CARTESIAN_POINT ( 'NONE',  ( -27.56211685706797709, 60.99999999999999289, -15.25056439471436676 ) ) ;
#8818=DIRECTION ( 'NONE',  ( -0.000000000000000000, 1.000000000000000000, -0.000000000000000000 ) ) ;
#8826=ORIENTED_EDGE ( 'NONE', *, *, #2723, .T. ) ;
#8827=CYLINDRICAL_SURFACE ( 'NONE', #5234, 1.500000000000001332 ) ;
#8829=AXIS2_PLACEMENT_3D ( 'NONE', #9147, #6074, #4706 ) ;
#8833=ADVANCED_FACE ( 'NONE', ( #1854, #4870 ), #612, .T. ) ;
#8835=VERTEX_POINT ( 'NONE', #5156 ) ;
#8839=ORIENTED_EDGE ( 'NONE', *, *, #6791, .T. ) ;
#8840=CIRCLE ( 'NONE', #4595, 37.00000000000000711 ) ;
#8850=ORIENTED_EDGE ( 'NONE', *, *, #51, .T. ) ;
#8855=ORIENTED_EDGE ( 'NONE', *, *, #3332, .F. ) ;
#8858=DIRECTION ( 'NONE',  ( 0.000000000000000000, 1.000000000000000000, 0.000000000000000000 ) ) ;
#8859=AXIS2_PLACEMENT_3D ( 'NONE', #9022, #2232, #2292 ) ;
#8865=DIRECTION ( 'NONE',  ( 0.000000000000000000, 0.000000000000000000, 1.000000000000000000 ) ) ;
#8868=DIRECTION ( 'NONE',  ( 0.000000000000000000, -0.000000000000000000, 1.000000000000000000 ) ) ;
#8872=AXIS2_PLACEMENT_3D ( 'NONE', #4745, #2495, #348 ) ;
#8875=CARTESIAN_POINT ( 'NONE',  ( -28.87459861216645862, 60.99999999999999289, -15.97678174684361707 ) ) ;
#8886=ORIENTED_EDGE ( 'NONE', *, *, #6780, .T. ) ;
#8889=EDGE_CURVE ( 'NONE', #9543, #2719, #2867, .T. ) ;
#8898=ORIENTED_EDGE ( 'NONE', *, *, #2231, .T. ) ;
#8901=DIRECTION ( 'NONE',  ( 0.000000000000000000, -1.000000000000000000, -0.000000000000000000 ) ) ;
#8916=CIRCLE ( 'NONE', #9548, 1.500000000000001332 ) ;
#8919=DIRECTION ( 'NONE',  ( 0.000000000000000000, 0.000000000000000000, 1.000000000000000000 ) ) ;
#8927=CARTESIAN_POINT ( 'NONE',  ( -8.106025752690484865, 61.92736406916336733, 36.79170325027453714 ) ) ;
#8929=DIRECTION ( 'NONE',  ( 0.000000000000000000, 0.000000000000000000, -1.000000000000000000 ) ) ;
#8935=VECTOR ( 'NONE', #3205, 1000.000000000000000 ) ;
#8939=ADVANCED_FACE ( 'NONE', ( #4371, #7374 ), #1299, .T. ) ;
#8943=EDGE_LOOP ( 'NONE', ( #424, #1684 ) ) ;
#8946=DIRECTION ( 'NONE',  ( 1.000000000000000000, 0.000000000000000000, 1.079383496163345602E-14 ) ) ;
#8950=CARTESIAN_POINT ( 'NONE',  ( 33.06426808735054124, 60.99999999999999289, 5.562309845534586294 ) ) ;
#8955=EDGE_LOOP ( 'NONE', ( #3376, #9041, #914, #3292, #2631 ) ) ;
#8961=DIRECTION ( 'NONE',  ( -0.000000000000000000, 1.000000000000000000, -0.000000000000000000 ) ) ;
#8962=DIRECTION ( 'NONE',  ( 0.000000000000000000, 0.000000000000000000, 1.000000000000000000 ) ) ;
#8967=ADVANCED_FACE ( 'NONE', ( #168 ), #5398, .T. ) ;
#8983=ORIENTED_EDGE ( 'NONE', *, *, #2617, .T. ) ;
#8988=AXIS2_PLACEMENT_3D ( 'NONE', #7730, #239, #2226 ) ;
#8999=VERTEX_POINT ( 'NONE', #6124 ) ;
#9012=CARTESIAN_POINT ( 'NONE',  ( 5.137569555611264605, 60.99999999999999289, 32.59762842694627949 ) ) ;
#9022=CARTESIAN_POINT ( 'NONE',  ( 0.000000000000000000, 58.99999999999999289, -37.00000000000000711 ) ) ;
#9023=CIRCLE ( 'NONE', #5861, 4.500000000000004441 ) ;
#9032=EDGE_CURVE ( 'NONE', #4372, #9299, #129, .T. ) ;
#9035=CARTESIAN_POINT ( 'NONE',  ( 3.429011037612588487E-15, 59.99999999999999289, 27.99999999999999289 ) ) ;
#9041=ORIENTED_EDGE ( 'NONE', *, *, #2240, .F. ) ;
#9062=ORIENTED_EDGE ( 'NONE', *, *, #3474, .T. ) ;
#9064=CIRCLE ( 'NONE', #3691, 31.49999999999999289 ) ;
#9068=CIRCLE ( 'NONE', #8117, 31.50000000000000000 ) ;
#9071=EDGE_LOOP ( 'NONE', ( #5089, #8648, #6650, #9 ) ) ;
#9080=FACE_OUTER_BOUND ( 'NONE', #1392, .T. ) ;
#9081=EDGE_LOOP ( 'NONE', ( #189, #8757, #1643, #846 ) ) ;
#9084=AXIS2_PLACEMENT_3D ( 'NONE', #3467, #1932, #368 ) ;
#9090=LINE ( 'NONE', #3293, #4942 ) ;
#9096=DIRECTION ( 'NONE',  ( 0.000000000000000000, 0.000000000000000000, 1.000000000000000000 ) ) ;
#9103=LINE ( 'NONE', #6015, #4207 ) ;
#9109=ORIENTED_EDGE ( 'NONE', *, *, #8287, .F. ) ;
#9120=DIRECTION ( 'NONE',  ( 0.000000000000000000, 0.000000000000000000, -1.000000000000000000 ) ) ;
#9122=EDGE_CURVE ( 'NONE', #4514, #5836, #1872, .T. ) ;
#9129=CARTESIAN_POINT ( 'NONE',  ( 33.06426808735054124, 60.99999999999999289, 5.562309845534586294 ) ) ;
#9134=DIRECTION ( 'NONE',  ( 0.000000000000000000, -1.000000000000000000, -0.000000000000000000 ) ) ;
#9144=ORIENTED_EDGE ( 'NONE', *, *, #2670, .T. ) ;
#9145=DIRECTION ( 'NONE',  ( 0.000000000000000000, 0.000000000000000000, -1.000000000000000000 ) ) ;
#9147=CARTESIAN_POINT ( 'NONE',  ( -5.137569555611031014, 61.99999999999999289, -32.59762842694632212 ) ) ;
#9156=DIRECTION ( 'NONE',  ( 0.000000000000000000, 0.000000000000000000, -1.000000000000000000 ) ) ;
#9157=CYLINDRICAL_SURFACE ( 'NONE', #1318, 34.50000000000000000 ) ;
#9158=EDGE_CURVE ( 'NONE', #5111, #7767, #4851, .T. ) ;
#9159=EDGE_CURVE ( 'NONE', #1536, #1139, #6565, .T. ) ;
#9175=VERTEX_POINT ( 'NONE', #3360 ) ;
#9180=DIRECTION ( 'NONE',  ( 0.000000000000000000, 0.000000000000000000, 1.000000000000000000 ) ) ;
#9187=CYLINDRICAL_SURFACE ( 'NONE', #2553, 1.500000000000001332 ) ;
#9191=CARTESIAN_POINT ( 'NONE',  ( 32.59762842694625817, 60.99999999999999289, -3.637569555611369854 ) ) ;
#9205=DIRECTION ( 'NONE',  ( -0.000000000000000000, -1.000000000000000000, -0.000000000000000000 ) ) ;
#9208=VECTOR ( 'NONE', #4252, 1000.000000000000000 ) ;
#9211=EDGE_LOOP ( 'NONE', ( #7392, #4506, #1727, #5595, #6824 ) ) ;
#9218=CARTESIAN_POINT ( 'NONE',  ( 5.562309845534588959, 69.99999999999998579, -33.06426808735054124 ) ) ;
#9221=FACE_BOUND ( 'NONE', #4212, .T. ) ;
#9228=DIRECTION ( 'NONE',  ( -0.000000000000000000, 1.000000000000000000, -0.000000000000000000 ) ) ;
#9230=CARTESIAN_POINT ( 'NONE',  ( -31.11591804390328164, 61.99999999999999289, 4.904043666719710259 ) ) ;
#9235=CARTESIAN_POINT ( 'NONE',  ( 36.28089590215267179, 61.98637676474528746, 8.721193672020515208 ) ) ;
#9240=CARTESIAN_POINT ( 'NONE',  ( 3.332326962091927580, 62.00000000000000711, -36.97859170863235789 ) ) ;
#9244=EDGE_CURVE ( 'NONE', #6026, #2210, #3962, .T. ) ;
#9246=EDGE_LOOP ( 'NONE', ( #5190, #5253, #402, #1399 ) ) ;
#9251=ORIENTED_EDGE ( 'NONE', *, *, #3957, .T. ) ;
#9258=FACE_OUTER_BOUND ( 'NONE', #4644, .T. ) ;
#9267=DIRECTION ( 'NONE',  ( 0.000000000000000000, 0.000000000000000000, -1.000000000000000000 ) ) ;
#9268=EDGE_CURVE ( 'NONE', #7767, #7682, #435, .T. ) ;
#9275=CARTESIAN_POINT ( 'NONE',  ( -5.562309845534584518, 69.99999999999998579, 35.56426808735054834 ) ) ;
#9277=DIRECTION ( 'NONE',  ( -0.000000000000000000, 1.000000000000000000, -0.000000000000000000 ) ) ;
#9280=EDGE_CURVE ( 'NONE', #5111, #326, #3893, .T. ) ;
#9283=ORIENTED_EDGE ( 'NONE', *, *, #4261, .F. ) ;
#9284=CARTESIAN_POINT ( 'NONE',  ( 7.214865095668090866, 61.84561525624321376, -37.26328141369675251 ) ) ;
#9285=CARTESIAN_POINT ( 'NONE',  ( 37.55900191124520404, 61.85658167520826822, 5.210294541070858543 ) ) ;
#9288=CARTESIAN_POINT ( 'NONE',  ( -37.19753653653384617, 61.85638901966269287, -7.362986651992473597 ) ) ;
#9292=CYLINDRICAL_SURFACE ( 'NONE', #1339, 34.49999999999999289 ) ;
#9296=DIRECTION ( 'NONE',  ( -1.000000000000000000, 0.000000000000000000, -3.083952846180987322E-15 ) ) ;
#9298=DIRECTION ( 'NONE',  ( 0.000000000000000000, 0.000000000000000000, 1.000000000000000000 ) ) ;
#9299=VERTEX_POINT ( 'NONE', #2454 ) ;
#9307=DIRECTION ( 'NONE',  ( 1.000000000000000000, 0.000000000000000000, 1.079383496163345602E-14 ) ) ;
#9311=EDGE_CURVE ( 'NONE', #7141, #5164, #9724, .T. ) ;
#9317=CIRCLE ( 'NONE', #5060, 2.499999999999998668 ) ;
#9324=CARTESIAN_POINT ( 'NONE',  ( -33.06426808735054124, 69.99999999999998579, -8.062309845534583630 ) ) ;
#9334=ORIENTED_EDGE ( 'NONE', *, *, #249, .T. ) ;
#9337=DIRECTION ( 'NONE',  ( 0.000000000000000000, 0.000000000000000000, 1.000000000000000000 ) ) ;
#9340=CIRCLE ( 'NONE', #671, 4.500000000000005329 ) ;
#9343=EDGE_CURVE ( 'NONE', #6468, #8122, #3949, .T. ) ;
#9353=AXIS2_PLACEMENT_3D ( 'NONE', #5318, #1749, #9120 ) ;
#9362=DIRECTION ( 'NONE',  ( -0.000000000000000000, 1.000000000000000000, -0.000000000000000000 ) ) ;
#9374=CARTESIAN_POINT ( 'NONE',  ( 37.19753653653384617, 61.85638901966269287, 7.362986651992473597 ) ) ;
#9377=CARTESIAN_POINT ( 'NONE',  ( 5.137569555611264605, 60.99999999999999289, 32.59762842694627949 ) ) ;
#9378=AXIS2_PLACEMENT_3D ( 'NONE', #3188, #886, #6890 ) ;
#9380=CARTESIAN_POINT ( 'NONE',  ( -37.01190402608325059, 62.00000000000000711, -3.384896555618068348 ) ) ;
#9383=AXIS2_PLACEMENT_3D ( 'NONE', #2153, #7359, #6510 ) ;
#9399=CARTESIAN_POINT ( 'NONE',  ( -33.06426808735054124, 60.99999999999999289, -10.06230984553459251 ) ) ;
#9405=ORIENTED_EDGE ( 'NONE', *, *, #1905, .T. ) ;
#9410=EDGE_CURVE ( 'NONE', #1736, #7319, #3496, .T. ) ;
#9414=AXIS2_PLACEMENT_3D ( 'NONE', #1469, #7505, #8443 ) ;
#9422=AXIS2_PLACEMENT_3D ( 'NONE', #3397, #630, #2097 ) ;
#9425=DIRECTION ( 'NONE',  ( -0.000000000000000000, -1.000000000000000000, -0.000000000000000000 ) ) ;
#9432=DIRECTION ( 'NONE',  ( 0.000000000000000000, 1.000000000000000000, 0.000000000000000000 ) ) ;
#9437=CARTESIAN_POINT ( 'NONE',  ( -36.64076086657617282, 61.94822636785970360, -8.307112375470062204 ) ) ;
#9439=ORIENTED_EDGE ( 'NONE', *, *, #8666, .T. ) ;
#9444=MANIFOLD_SOLID_BREP ( 'Cut-Extrude5', #3898 ) ;
#9450=LINE ( 'NONE', #9399, #1259 ) ;
#9455=ORIENTED_EDGE ( 'NONE', *, *, #5225, .T. ) ;
#9458=DIRECTION ( 'NONE',  ( 1.000000000000000000, 0.000000000000000000, -1.224646799147353207E-16 ) ) ;
#9463=ORIENTED_EDGE ( 'NONE', *, *, #2015, .F. ) ;
#9468=CYLINDRICAL_SURFACE ( 'NONE', #5387, 2.500000000000002220 ) ;
#9469=DIRECTION ( 'NONE',  ( 0.000000000000000000, 1.000000000000000000, 0.000000000000000000 ) ) ;
#9474=DIRECTION ( 'NONE',  ( 0.000000000000000000, -1.000000000000000000, 0.000000000000000000 ) ) ;
#9478=CARTESIAN_POINT ( 'NONE',  ( 33.06426808735054124, 61.99999999999999289, 10.06230984553459251 ) ) ;
#9479=CARTESIAN_POINT ( 'NONE',  ( 0.000000000000000000, 0.000000000000000000, 0.000000000000000000 ) ) ;
#9482=FACE_BOUND ( 'NONE', #57, .T. ) ;
#9485=CARTESIAN_POINT ( 'NONE',  ( 0.000000000000000000, 59.99999999999999289, -27.99999999999999289 ) ) ;
#9505=CARTESIAN_POINT ( 'NONE',  ( 33.06426808735054124, 60.99999999999999289, 10.06230984553459251 ) ) ;
#9506=AXIS2_PLACEMENT_3D ( 'NONE', #792, #3803, #9096 ) ;
#9517=ORIENTED_EDGE ( 'NONE', *, *, #1954, .F. ) ;
#9530=DIRECTION ( 'NONE',  ( -0.000000000000000000, -1.000000000000000000, -0.000000000000000000 ) ) ;
#9534=AXIS2_PLACEMENT_3D ( 'NONE', #8280, #2940, #5952 ) ;
#9537=EDGE_CURVE ( 'NONE', #4366, #4372, #6409, .T. ) ;
#9543=VERTEX_POINT ( 'NONE', #98 ) ;
#9548=AXIS2_PLACEMENT_3D ( 'NONE', #4707, #7713, #8505 ) ;
#9553=AXIS2_PLACEMENT_3D ( 'NONE', #315, #6325, #5548 ) ;
#9554=ORIENTED_EDGE ( 'NONE', *, *, #4513, .F. ) ;
#9555=DIRECTION ( 'NONE',  ( 0.000000000000000000, 0.000000000000000000, -1.000000000000000000 ) ) ;
#9564=AXIS2_PLACEMENT_3D ( 'NONE', #7691, #7077, #5102 ) ;
#9585=DIRECTION ( 'NONE',  ( 0.000000000000000000, 1.000000000000000000, 0.000000000000000000 ) ) ;
#9595=ORIENTED_EDGE ( 'NONE', *, *, #7697, .T. ) ;
#9603=CARTESIAN_POINT ( 'NONE',  ( -5.562309845534701758, 61.99999999999999289, 33.06426808735052703 ) ) ;
#9604=ORIENTED_EDGE ( 'NONE', *, *, #1305, .F. ) ;
#9607=FACE_BOUND ( 'NONE', #8707, .T. ) ;
#9610=DIRECTION ( 'NONE',  ( 0.000000000000000000, 0.000000000000000000, -1.000000000000000000 ) ) ;
#9614=VERTEX_POINT ( 'NONE', #8187 ) ;
#9617=CIRCLE ( 'NONE', #8680, 31.50000000000000000 ) ;
#9618=AXIS2_PLACEMENT_3D ( 'NONE', #1710, #2393, #4727 ) ;
#9621=CYLINDRICAL_SURFACE ( 'NONE', #3865, 31.50000000000000000 ) ;
#9623=CARTESIAN_POINT ( 'NONE',  ( -4.904043666719616112, 60.99999999999999289, -31.11591804390330651 ) ) ;
#9641=ORIENTED_EDGE ( 'NONE', *, *, #9311, .F. ) ;
#9643=DIRECTION ( 'NONE',  ( 0.000000000000000000, -1.000000000000000000, 0.000000000000000000 ) ) ;
#9649=EDGE_LOOP ( 'NONE', ( #6206, #1703, #765, #9439, #36, #277 ) ) ;
#9651=ORIENTED_EDGE ( 'NONE', *, *, #1386, .T. ) ;
#9654=CARTESIAN_POINT ( 'NONE',  ( 0.000000000000000000, 0.000000000000000000, 0.000000000000000000 ) ) ;
#9655=CARTESIAN_POINT ( 'NONE',  ( 5.562309845534588959, 59.99999999999999289, -33.06426808735054124 ) ) ;
#9656=AXIS2_PLACEMENT_3D ( 'NONE', #3766, #6914, #6128 ) ;
#9668=CIRCLE ( 'NONE', #1159, 4.500000000000005329 ) ;
#9675=CARTESIAN_POINT ( 'NONE',  ( -5.562309845534701758, 61.83753588906734677, 37.56426808735052703 ) ) ;
#9689=ADVANCED_FACE ( 'NONE', ( #4641 ), #7693, .T. ) ;
#9710=AXIS2_PLACEMENT_3D ( 'NONE', #8227, #1371, #4482 ) ;
#9711=AXIS2_PLACEMENT_3D ( 'NONE', #8875, #3683, #2985 ) ;
#9713=CARTESIAN_POINT ( 'NONE',  ( -5.562309845534584518, 59.99999999999999289, 33.06426808735054124 ) ) ;
#9714=VERTEX_POINT ( 'NONE', #8634 ) ;
#9720=DIRECTION ( 'NONE',  ( 0.000000000000000000, 1.000000000000000000, 0.000000000000000000 ) ) ;
#9724=CIRCLE ( 'NONE', #6871, 3.000000000000002665 ) ;
#9726=ORIENTED_EDGE ( 'NONE', *, *, #3649, .T. ) ;
#9738=CARTESIAN_POINT ( 'NONE',  ( 33.06426808735054124, 59.99999999999999289, 5.562309845534586294 ) ) ;
#9746=ADVANCED_FACE ( 'NONE', ( #383 ), #9468, .F. ) ;
#9779=COLOUR_RGB('Sky Blue',0.24,0.69,0.87);
#9780=FILL_AREA_STYLE_COLOUR('',#9779);
#9781=FILL_AREA_STYLE('',(#9780));
#9782=SURFACE_STYLE_FILL_AREA(#9781);
#9783=SURFACE_SIDE_STYLE('',(#9782));
#9784=SURFACE_STYLE_USAGE(.BOTH.,#9783);
#9785=PRESENTATION_STYLE_ASSIGNMENT((#9784));
ENDSEC;
END-ISO-10303-21;
